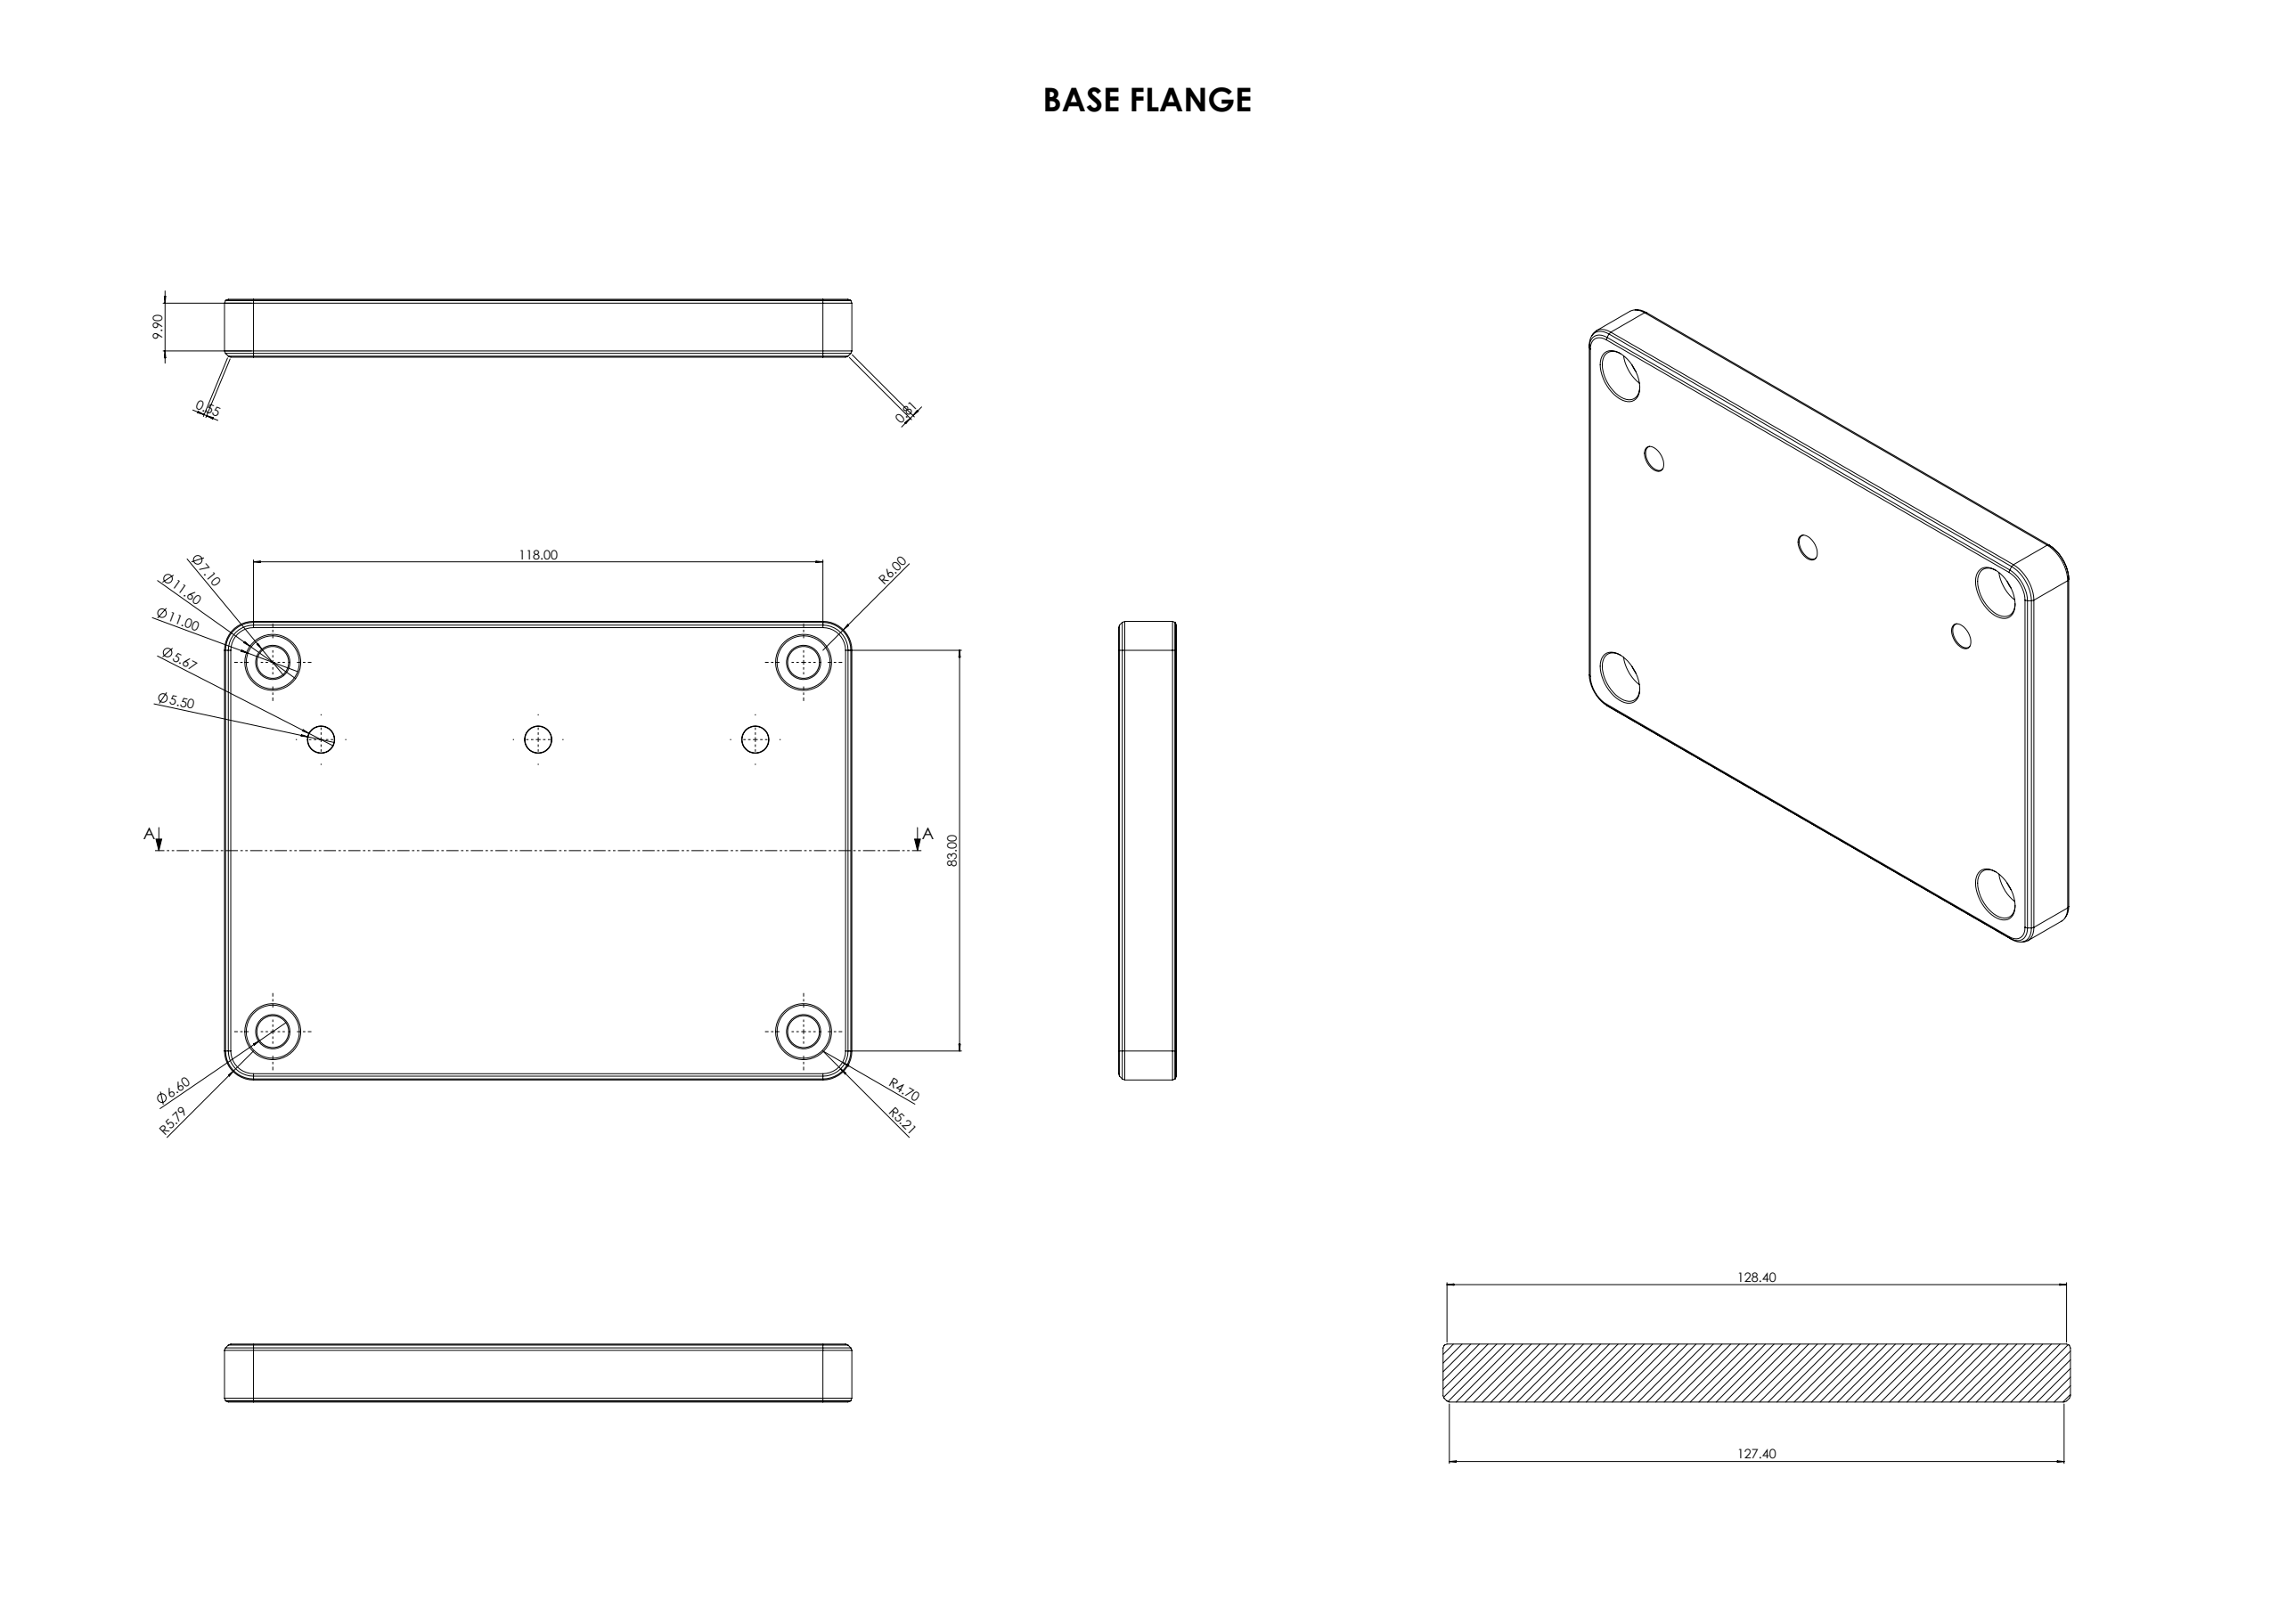
ISO-10303-21;
HEADER;
/* Generated by software containing ST-Developer
 * from STEP Tools, Inc. (www.steptools.com) 
 */

FILE_DESCRIPTION(
/* description */ (''),
/* implementation_level */ '2;1');

FILE_NAME(
/* name */ '01_Base_Flange.step',
/* time_stamp */ '2026-10-19T22:59:19-07:00',
/* author */ (''),
/* organization */ (''),
/* preprocessor_version */ 'ST-DEVELOPER v20.2',
/* originating_system */ 'Autodesk Translation Framework v15.15.0.0',
/* authorisation */ '');

FILE_SCHEMA (('AUTOMOTIVE_DESIGN { 1 0 10303 214 3 1 1 }'));
ENDSEC;

DATA;
#10=MECHANICAL_DESIGN_GEOMETRIC_PRESENTATION_REPRESENTATION('',(#911),#53650);
#879=SHAPE_REPRESENTATION_RELATIONSHIP('SRR','None',#53724,#895);
#895=ADVANCED_BREP_SHAPE_REPRESENTATION('',(#927),#53634);
#911=STYLED_ITEM('',(#53937),#927);
#927=MANIFOLD_SOLID_BREP('Base Flange',#23303);
#943=CYLINDRICAL_SURFACE('',#23543,0.6);
#944=CYLINDRICAL_SURFACE('',#23546,0.6);
#945=CYLINDRICAL_SURFACE('',#23599,0.55);
#946=CYLINDRICAL_SURFACE('',#23604,0.55);
#947=CYLINDRICAL_SURFACE('',#23609,0.55);
#948=CYLINDRICAL_SURFACE('',#23614,0.55);
#949=CYLINDRICAL_SURFACE('',#23619,0.5);
#950=CYLINDRICAL_SURFACE('',#23624,0.5);
#951=CYLINDRICAL_SURFACE('',#23629,0.5);
#952=CYLINDRICAL_SURFACE('',#23633,0.275);
#953=CYLINDRICAL_SURFACE('',#23640,0.275);
#954=CYLINDRICAL_SURFACE('',#23647,0.275);
#955=CYLINDRICAL_SURFACE('',#23654,0.33);
#956=CYLINDRICAL_SURFACE('',#23661,0.33);
#957=CYLINDRICAL_SURFACE('',#23668,0.33);
#958=CYLINDRICAL_SURFACE('',#23675,0.33);
#959=CYLINDRICAL_SURFACE('',#23683,0.6);
#960=CYLINDRICAL_SURFACE('',#23684,0.6);
#1277=FACE_BOUND('',#3577,.T.);
#1278=FACE_BOUND('',#3578,.T.);
#1279=FACE_BOUND('',#3579,.T.);
#1280=FACE_BOUND('',#3580,.T.);
#1281=FACE_BOUND('',#3581,.T.);
#1282=FACE_BOUND('',#3582,.T.);
#1283=FACE_BOUND('',#3583,.T.);
#1284=FACE_BOUND('',#3612,.T.);
#1285=FACE_BOUND('',#3613,.T.);
#1286=FACE_BOUND('',#3614,.T.);
#1287=FACE_BOUND('',#3615,.T.);
#1288=FACE_BOUND('',#3616,.T.);
#1289=FACE_BOUND('',#3617,.T.);
#1290=FACE_BOUND('',#3618,.T.);
#1291=FACE_BOUND('',#3648,.T.);
#1292=FACE_BOUND('',#3653,.T.);
#1293=FACE_BOUND('',#3658,.T.);
#1294=FACE_BOUND('',#3663,.T.);
#1295=FACE_BOUND('',#3668,.T.);
#1296=FACE_BOUND('',#3673,.T.);
#1297=FACE_BOUND('',#3678,.T.);
#1448=PLANE('',#23501);
#1449=PLANE('',#23505);
#1450=PLANE('',#23509);
#1451=PLANE('',#23513);
#1452=PLANE('',#23514);
#1453=PLANE('',#23517);
#1454=PLANE('',#23520);
#1455=PLANE('',#23530);
#1456=PLANE('',#23533);
#1457=PLANE('',#23537);
#1458=PLANE('',#23541);
#1459=PLANE('',#23542);
#1460=PLANE('',#23545);
#1461=PLANE('',#23548);
#1462=PLANE('',#23550);
#1463=PLANE('',#23551);
#1464=PLANE('',#23555);
#1465=PLANE('',#23559);
#1466=PLANE('',#23563);
#1467=PLANE('',#23569);
#1468=PLANE('',#23572);
#1469=PLANE('',#23573);
#1470=PLANE('',#23581);
#1471=PLANE('',#23583);
#1472=PLANE('',#23585);
#1473=PLANE('',#23589);
#1474=PLANE('',#23594);
#1475=PLANE('',#23637);
#1476=PLANE('',#23644);
#1477=PLANE('',#23651);
#1478=PLANE('',#23658);
#1479=PLANE('',#23665);
#1480=PLANE('',#23672);
#1481=PLANE('',#23679);
#1482=PLANE('',#23680);
#1483=PLANE('',#23682);
#1484=PLANE('',#23685);
#2236=FACE_OUTER_BOUND('',#3564,.T.);
#2237=FACE_OUTER_BOUND('',#3565,.T.);
#2238=FACE_OUTER_BOUND('',#3566,.T.);
#2239=FACE_OUTER_BOUND('',#3567,.T.);
#2240=FACE_OUTER_BOUND('',#3568,.T.);
#2241=FACE_OUTER_BOUND('',#3569,.T.);
#2242=FACE_OUTER_BOUND('',#3570,.T.);
#2243=FACE_OUTER_BOUND('',#3571,.T.);
#2244=FACE_OUTER_BOUND('',#3572,.T.);
#2245=FACE_OUTER_BOUND('',#3573,.T.);
#2246=FACE_OUTER_BOUND('',#3574,.T.);
#2247=FACE_OUTER_BOUND('',#3575,.T.);
#2248=FACE_OUTER_BOUND('',#3576,.T.);
#2249=FACE_OUTER_BOUND('',#3584,.T.);
#2250=FACE_OUTER_BOUND('',#3585,.T.);
#2251=FACE_OUTER_BOUND('',#3586,.T.);
#2252=FACE_OUTER_BOUND('',#3587,.T.);
#2253=FACE_OUTER_BOUND('',#3588,.T.);
#2254=FACE_OUTER_BOUND('',#3589,.T.);
#2255=FACE_OUTER_BOUND('',#3590,.T.);
#2256=FACE_OUTER_BOUND('',#3591,.T.);
#2257=FACE_OUTER_BOUND('',#3592,.T.);
#2258=FACE_OUTER_BOUND('',#3593,.T.);
#2259=FACE_OUTER_BOUND('',#3594,.T.);
#2260=FACE_OUTER_BOUND('',#3595,.T.);
#2261=FACE_OUTER_BOUND('',#3596,.T.);
#2262=FACE_OUTER_BOUND('',#3597,.T.);
#2263=FACE_OUTER_BOUND('',#3598,.T.);
#2264=FACE_OUTER_BOUND('',#3599,.T.);
#2265=FACE_OUTER_BOUND('',#3600,.T.);
#2266=FACE_OUTER_BOUND('',#3601,.T.);
#2267=FACE_OUTER_BOUND('',#3602,.T.);
#2268=FACE_OUTER_BOUND('',#3603,.T.);
#2269=FACE_OUTER_BOUND('',#3604,.T.);
#2270=FACE_OUTER_BOUND('',#3605,.T.);
#2271=FACE_OUTER_BOUND('',#3606,.T.);
#2272=FACE_OUTER_BOUND('',#3607,.T.);
#2273=FACE_OUTER_BOUND('',#3608,.T.);
#2274=FACE_OUTER_BOUND('',#3609,.T.);
#2275=FACE_OUTER_BOUND('',#3610,.T.);
#2276=FACE_OUTER_BOUND('',#3611,.T.);
#2277=FACE_OUTER_BOUND('',#3619,.T.);
#2278=FACE_OUTER_BOUND('',#3620,.T.);
#2279=FACE_OUTER_BOUND('',#3621,.T.);
#2280=FACE_OUTER_BOUND('',#3622,.T.);
#2281=FACE_OUTER_BOUND('',#3623,.T.);
#2282=FACE_OUTER_BOUND('',#3624,.T.);
#2283=FACE_OUTER_BOUND('',#3625,.T.);
#2284=FACE_OUTER_BOUND('',#3626,.T.);
#2285=FACE_OUTER_BOUND('',#3627,.T.);
#2286=FACE_OUTER_BOUND('',#3628,.T.);
#2287=FACE_OUTER_BOUND('',#3629,.T.);
#2288=FACE_OUTER_BOUND('',#3630,.T.);
#2289=FACE_OUTER_BOUND('',#3631,.T.);
#2290=FACE_OUTER_BOUND('',#3632,.T.);
#2291=FACE_OUTER_BOUND('',#3633,.T.);
#2292=FACE_OUTER_BOUND('',#3634,.T.);
#2293=FACE_OUTER_BOUND('',#3635,.T.);
#2294=FACE_OUTER_BOUND('',#3636,.T.);
#2295=FACE_OUTER_BOUND('',#3637,.T.);
#2296=FACE_OUTER_BOUND('',#3638,.T.);
#2297=FACE_OUTER_BOUND('',#3639,.T.);
#2298=FACE_OUTER_BOUND('',#3640,.T.);
#2299=FACE_OUTER_BOUND('',#3641,.T.);
#2300=FACE_OUTER_BOUND('',#3642,.T.);
#2301=FACE_OUTER_BOUND('',#3643,.T.);
#2302=FACE_OUTER_BOUND('',#3644,.T.);
#2303=FACE_OUTER_BOUND('',#3645,.T.);
#2304=FACE_OUTER_BOUND('',#3646,.T.);
#2305=FACE_OUTER_BOUND('',#3647,.T.);
#2306=FACE_OUTER_BOUND('',#3649,.T.);
#2307=FACE_OUTER_BOUND('',#3650,.T.);
#2308=FACE_OUTER_BOUND('',#3651,.T.);
#2309=FACE_OUTER_BOUND('',#3652,.T.);
#2310=FACE_OUTER_BOUND('',#3654,.T.);
#2311=FACE_OUTER_BOUND('',#3655,.T.);
#2312=FACE_OUTER_BOUND('',#3656,.T.);
#2313=FACE_OUTER_BOUND('',#3657,.T.);
#2314=FACE_OUTER_BOUND('',#3659,.T.);
#2315=FACE_OUTER_BOUND('',#3660,.T.);
#2316=FACE_OUTER_BOUND('',#3661,.T.);
#2317=FACE_OUTER_BOUND('',#3662,.T.);
#2318=FACE_OUTER_BOUND('',#3664,.T.);
#2319=FACE_OUTER_BOUND('',#3665,.T.);
#2320=FACE_OUTER_BOUND('',#3666,.T.);
#2321=FACE_OUTER_BOUND('',#3667,.T.);
#2322=FACE_OUTER_BOUND('',#3669,.T.);
#2323=FACE_OUTER_BOUND('',#3670,.T.);
#2324=FACE_OUTER_BOUND('',#3671,.T.);
#2325=FACE_OUTER_BOUND('',#3672,.T.);
#2326=FACE_OUTER_BOUND('',#3674,.T.);
#2327=FACE_OUTER_BOUND('',#3675,.T.);
#2328=FACE_OUTER_BOUND('',#3676,.T.);
#2329=FACE_OUTER_BOUND('',#3677,.T.);
#2330=FACE_OUTER_BOUND('',#3679,.T.);
#2331=FACE_OUTER_BOUND('',#3680,.T.);
#2332=FACE_OUTER_BOUND('',#3681,.T.);
#2333=FACE_OUTER_BOUND('',#3682,.T.);
#2334=FACE_OUTER_BOUND('',#3683,.T.);
#2335=FACE_OUTER_BOUND('',#3684,.T.);
#3564=EDGE_LOOP('',(#15067,#15068,#15069,#15070));
#3565=EDGE_LOOP('',(#15071,#15072,#15073,#15074));
#3566=EDGE_LOOP('',(#15075,#15076,#15077,#15078));
#3567=EDGE_LOOP('',(#15079,#15080,#15081,#15082));
#3568=EDGE_LOOP('',(#15083,#15084,#15085,#15086));
#3569=EDGE_LOOP('',(#15087,#15088,#15089,#15090));
#3570=EDGE_LOOP('',(#15091,#15092,#15093,#15094));
#3571=EDGE_LOOP('',(#15095,#15096,#15097,#15098));
#3572=EDGE_LOOP('',(#15099,#15100,#15101,#15102));
#3573=EDGE_LOOP('',(#15103,#15104,#15105,#15106));
#3574=EDGE_LOOP('',(#15107,#15108,#15109,#15110));
#3575=EDGE_LOOP('',(#15111,#15112,#15113,#15114));
#3576=EDGE_LOOP('',(#15115,#15116,#15117,#15118,#15119,#15120,#15121,#15122));
#3577=EDGE_LOOP('',(#15123));
#3578=EDGE_LOOP('',(#15124));
#3579=EDGE_LOOP('',(#15125));
#3580=EDGE_LOOP('',(#15126));
#3581=EDGE_LOOP('',(#15127));
#3582=EDGE_LOOP('',(#15128));
#3583=EDGE_LOOP('',(#15129));
#3584=EDGE_LOOP('',(#15130,#15131,#15132,#15133));
#3585=EDGE_LOOP('',(#15134,#15135,#15136,#15137));
#3586=EDGE_LOOP('',(#15138,#15139,#15140,#15141));
#3587=EDGE_LOOP('',(#15142,#15143,#15144,#15145));
#3588=EDGE_LOOP('',(#15146,#15147,#15148,#15149));
#3589=EDGE_LOOP('',(#15150,#15151,#15152,#15153));
#3590=EDGE_LOOP('',(#15154,#15155,#15156,#15157));
#3591=EDGE_LOOP('',(#15158,#15159,#15160,#15161));
#3592=EDGE_LOOP('',(#15162,#15163,#15164,#15165));
#3593=EDGE_LOOP('',(#15166,#15167,#15168,#15169));
#3594=EDGE_LOOP('',(#15170,#15171,#15172,#15173));
#3595=EDGE_LOOP('',(#15174,#15175,#15176,#15177));
#3596=EDGE_LOOP('',(#15178,#15179,#15180,#15181));
#3597=EDGE_LOOP('',(#15182,#15183,#15184,#15185));
#3598=EDGE_LOOP('',(#15186,#15187,#15188,#15189));
#3599=EDGE_LOOP('',(#15190,#15191,#15192,#15193));
#3600=EDGE_LOOP('',(#15194,#15195,#15196,#15197));
#3601=EDGE_LOOP('',(#15198,#15199,#15200,#15201));
#3602=EDGE_LOOP('',(#15202,#15203,#15204,#15205));
#3603=EDGE_LOOP('',(#15206,#15207,#15208,#15209));
#3604=EDGE_LOOP('',(#15210,#15211,#15212,#15213));
#3605=EDGE_LOOP('',(#15214,#15215,#15216,#15217));
#3606=EDGE_LOOP('',(#15218,#15219,#15220,#15221));
#3607=EDGE_LOOP('',(#15222,#15223,#15224,#15225));
#3608=EDGE_LOOP('',(#15226,#15227,#15228,#15229));
#3609=EDGE_LOOP('',(#15230,#15231,#15232,#15233));
#3610=EDGE_LOOP('',(#15234,#15235,#15236,#15237));
#3611=EDGE_LOOP('',(#15238,#15239,#15240,#15241,#15242,#15243,#15244,#15245));
#3612=EDGE_LOOP('',(#15246));
#3613=EDGE_LOOP('',(#15247));
#3614=EDGE_LOOP('',(#15248));
#3615=EDGE_LOOP('',(#15249));
#3616=EDGE_LOOP('',(#15250));
#3617=EDGE_LOOP('',(#15251));
#3618=EDGE_LOOP('',(#15252));
#3619=EDGE_LOOP('',(#15253,#15254,#15255,#15256));
#3620=EDGE_LOOP('',(#15257,#15258,#15259,#15260));
#3621=EDGE_LOOP('',(#15261,#15262,#15263,#15264));
#3622=EDGE_LOOP('',(#15265,#15266,#15267,#15268));
#3623=EDGE_LOOP('',(#15269,#15270,#15271,#15272));
#3624=EDGE_LOOP('',(#15273,#15274,#15275,#15276));
#3625=EDGE_LOOP('',(#15277,#15278,#15279,#15280));
#3626=EDGE_LOOP('',(#15281,#15282,#15283,#15284));
#3627=EDGE_LOOP('',(#15285,#15286,#15287,#15288));
#3628=EDGE_LOOP('',(#15289,#15290,#15291,#15292));
#3629=EDGE_LOOP('',(#15293,#15294,#15295,#15296));
#3630=EDGE_LOOP('',(#15297,#15298,#15299,#15300,#15301));
#3631=EDGE_LOOP('',(#15302,#15303,#15304,#15305,#15306));
#3632=EDGE_LOOP('',(#15307,#15308,#15309,#15310,#15311));
#3633=EDGE_LOOP('',(#15312,#15313,#15314,#15315,#15316));
#3634=EDGE_LOOP('',(#15317,#15318,#15319,#15320,#15321));
#3635=EDGE_LOOP('',(#15322,#15323,#15324,#15325,#15326));
#3636=EDGE_LOOP('',(#15327,#15328,#15329,#15330,#15331));
#3637=EDGE_LOOP('',(#15332,#15333,#15334,#15335,#15336));
#3638=EDGE_LOOP('',(#15337,#15338,#15339,#15340,#15341));
#3639=EDGE_LOOP('',(#15342,#15343,#15344,#15345,#15346));
#3640=EDGE_LOOP('',(#15347,#15348,#15349,#15350,#15351));
#3641=EDGE_LOOP('',(#15352,#15353,#15354,#15355,#15356));
#3642=EDGE_LOOP('',(#15357,#15358,#15359,#15360,#15361));
#3643=EDGE_LOOP('',(#15362,#15363,#15364,#15365,#15366));
#3644=EDGE_LOOP('',(#15367,#15368,#15369,#15370));
#3645=EDGE_LOOP('',(#15371,#15372,#15373,#15374));
#3646=EDGE_LOOP('',(#15375,#15376,#15377,#15378));
#3647=EDGE_LOOP('',(#15379));
#3648=EDGE_LOOP('',(#15380));
#3649=EDGE_LOOP('',(#15381,#15382,#15383,#15384));
#3650=EDGE_LOOP('',(#15385,#15386,#15387,#15388));
#3651=EDGE_LOOP('',(#15389,#15390,#15391,#15392));
#3652=EDGE_LOOP('',(#15393));
#3653=EDGE_LOOP('',(#15394));
#3654=EDGE_LOOP('',(#15395,#15396,#15397,#15398));
#3655=EDGE_LOOP('',(#15399,#15400,#15401,#15402));
#3656=EDGE_LOOP('',(#15403,#15404,#15405,#15406));
#3657=EDGE_LOOP('',(#15407));
#3658=EDGE_LOOP('',(#15408));
#3659=EDGE_LOOP('',(#15409,#15410,#15411,#15412));
#3660=EDGE_LOOP('',(#15413,#15414,#15415,#15416));
#3661=EDGE_LOOP('',(#15417,#15418,#15419,#15420));
#3662=EDGE_LOOP('',(#15421));
#3663=EDGE_LOOP('',(#15422));
#3664=EDGE_LOOP('',(#15423,#15424,#15425,#15426));
#3665=EDGE_LOOP('',(#15427,#15428,#15429,#15430));
#3666=EDGE_LOOP('',(#15431,#15432,#15433,#15434));
#3667=EDGE_LOOP('',(#15435));
#3668=EDGE_LOOP('',(#15436));
#3669=EDGE_LOOP('',(#15437,#15438,#15439,#15440));
#3670=EDGE_LOOP('',(#15441,#15442,#15443,#15444));
#3671=EDGE_LOOP('',(#15445,#15446,#15447,#15448));
#3672=EDGE_LOOP('',(#15449));
#3673=EDGE_LOOP('',(#15450));
#3674=EDGE_LOOP('',(#15451,#15452,#15453,#15454));
#3675=EDGE_LOOP('',(#15455,#15456,#15457,#15458));
#3676=EDGE_LOOP('',(#15459,#15460,#15461,#15462));
#3677=EDGE_LOOP('',(#15463));
#3678=EDGE_LOOP('',(#15464));
#3679=EDGE_LOOP('',(#15465,#15466,#15467,#15468));
#3680=EDGE_LOOP('',(#15469,#15470,#15471,#15472));
#3681=EDGE_LOOP('',(#15473,#15474,#15475,#15476));
#3682=EDGE_LOOP('',(#15477,#15478,#15479,#15480));
#3683=EDGE_LOOP('',(#15481,#15482,#15483,#15484));
#3684=EDGE_LOOP('',(#15485,#15486,#15487,#15488));
#5063=CIRCLE('',#23499,0.521213203435596);
#5064=CIRCLE('',#23500,0.47);
#5065=CIRCLE('',#23503,0.521213203435596);
#5066=CIRCLE('',#23504,0.47);
#5067=CIRCLE('',#23507,0.521213203435596);
#5068=CIRCLE('',#23508,0.47);
#5069=CIRCLE('',#23511,0.521213203435596);
#5070=CIRCLE('',#23512,0.47);
#5071=CIRCLE('',#23516,0.578786796564404);
#5072=CIRCLE('',#23519,0.578786796564404);
#5073=CIRCLE('',#23521,0.58);
#5074=CIRCLE('',#23522,0.58);
#5075=CIRCLE('',#23523,0.283333333333333);
#5076=CIRCLE('',#23524,0.283333333333333);
#5077=CIRCLE('',#23525,0.283333333333333);
#5078=CIRCLE('',#23526,0.58);
#5079=CIRCLE('',#23527,0.58);
#5080=CIRCLE('',#23529,0.6);
#5081=CIRCLE('',#23532,0.6);
#5082=CIRCLE('',#23535,0.578786796564404);
#5083=CIRCLE('',#23536,0.6);
#5084=CIRCLE('',#23539,0.578786796564404);
#5085=CIRCLE('',#23540,0.6);
#5086=CIRCLE('',#23544,0.6);
#5087=CIRCLE('',#23547,0.6);
#5088=CIRCLE('',#23553,0.571213203435596);
#5089=CIRCLE('',#23554,0.52);
#5090=CIRCLE('',#23557,0.571213203435596);
#5091=CIRCLE('',#23558,0.52);
#5092=CIRCLE('',#23561,0.571213203435596);
#5093=CIRCLE('',#23562,0.52);
#5094=CIRCLE('',#23565,0.571213203435596);
#5095=CIRCLE('',#23566,0.52);
#5096=CIRCLE('',#23568,0.578786796564404);
#5097=CIRCLE('',#23571,0.578786796564404);
#5098=CIRCLE('',#23574,0.53);
#5099=CIRCLE('',#23575,0.53);
#5100=CIRCLE('',#23576,0.338333333333333);
#5101=CIRCLE('',#23577,0.338333333333333);
#5102=CIRCLE('',#23578,0.338333333333333);
#5103=CIRCLE('',#23579,0.338333333333333);
#5104=CIRCLE('',#23580,0.53);
#5105=CIRCLE('',#23587,0.578786796564404);
#5106=CIRCLE('',#23588,0.6);
#5107=CIRCLE('',#23591,0.578786796564404);
#5108=CIRCLE('',#23592,0.6);
#5109=CIRCLE('',#23597,0.55);
#5110=CIRCLE('',#23598,0.55);
#5111=CIRCLE('',#23600,0.55);
#5112=CIRCLE('',#23602,0.55);
#5113=CIRCLE('',#23603,0.55);
#5114=CIRCLE('',#23605,0.55);
#5115=CIRCLE('',#23607,0.55);
#5116=CIRCLE('',#23608,0.55);
#5117=CIRCLE('',#23610,0.55);
#5118=CIRCLE('',#23612,0.55);
#5119=CIRCLE('',#23613,0.55);
#5120=CIRCLE('',#23615,0.55);
#5121=CIRCLE('',#23617,0.5);
#5122=CIRCLE('',#23618,0.5);
#5123=CIRCLE('',#23620,0.5);
#5124=CIRCLE('',#23622,0.5);
#5125=CIRCLE('',#23623,0.5);
#5126=CIRCLE('',#23625,0.5);
#5127=CIRCLE('',#23627,0.5);
#5128=CIRCLE('',#23628,0.5);
#5129=CIRCLE('',#23630,0.5);
#5130=CIRCLE('',#23632,0.275);
#5131=CIRCLE('',#23634,0.275);
#5132=CIRCLE('',#23636,0.3);
#5133=CIRCLE('',#23639,0.275);
#5134=CIRCLE('',#23641,0.275);
#5135=CIRCLE('',#23643,0.3);
#5136=CIRCLE('',#23646,0.275);
#5137=CIRCLE('',#23648,0.275);
#5138=CIRCLE('',#23650,0.3);
#5139=CIRCLE('',#23653,0.33);
#5140=CIRCLE('',#23655,0.33);
#5141=CIRCLE('',#23657,0.355);
#5142=CIRCLE('',#23660,0.33);
#5143=CIRCLE('',#23662,0.33);
#5144=CIRCLE('',#23664,0.355);
#5145=CIRCLE('',#23667,0.33);
#5146=CIRCLE('',#23669,0.33);
#5147=CIRCLE('',#23671,0.355);
#5148=CIRCLE('',#23674,0.33);
#5149=CIRCLE('',#23676,0.33);
#5150=CIRCLE('',#23678,0.355);
#5852=LINE('',#31820,#7697);
#5853=LINE('',#31824,#7698);
#5854=LINE('',#31829,#7699);
#5855=LINE('',#31830,#7700);
#5856=LINE('',#31831,#7701);
#5857=LINE('',#31835,#7702);
#5858=LINE('',#31841,#7703);
#5859=LINE('',#31842,#7704);
#5860=LINE('',#31843,#7705);
#5861=LINE('',#31847,#7706);
#5862=LINE('',#31853,#7707);
#5863=LINE('',#31854,#7708);
#5864=LINE('',#31855,#7709);
#5865=LINE('',#31859,#7710);
#5866=LINE('',#31863,#7711);
#5867=LINE('',#31864,#7712);
#5868=LINE('',#31867,#7713);
#5869=LINE('',#31869,#7714);
#5870=LINE('',#31870,#7715);
#5871=LINE('',#31873,#7716);
#5872=LINE('',#31877,#7717);
#5873=LINE('',#31878,#7718);
#5874=LINE('',#31881,#7719);
#5875=LINE('',#31900,#7720);
#5876=LINE('',#31902,#7721);
#5877=LINE('',#31906,#7722);
#5878=LINE('',#31907,#7723);
#5879=LINE('',#31910,#7724);
#5880=LINE('',#31914,#7725);
#5881=LINE('',#31915,#7726);
#5882=LINE('',#31919,#7727);
#5883=LINE('',#31925,#7728);
#5884=LINE('',#31926,#7729);
#5885=LINE('',#31927,#7730);
#5886=LINE('',#31931,#7731);
#5887=LINE('',#31935,#7732);
#5888=LINE('',#31936,#7733);
#5889=LINE('',#31939,#7734);
#5890=LINE('',#31941,#7735);
#5891=LINE('',#31942,#7736);
#5892=LINE('',#31945,#7737);
#5893=LINE('',#31949,#7738);
#5894=LINE('',#31950,#7739);
#5895=LINE('',#31953,#7740);
#5896=LINE('',#31956,#7741);
#5897=LINE('',#31957,#7742);
#5898=LINE('',#31959,#7743);
#5899=LINE('',#31964,#7744);
#5900=LINE('',#31966,#7745);
#5901=LINE('',#31968,#7746);
#5902=LINE('',#31969,#7747);
#5903=LINE('',#31973,#7748);
#5904=LINE('',#31979,#7749);
#5905=LINE('',#31980,#7750);
#5906=LINE('',#31981,#7751);
#5907=LINE('',#31985,#7752);
#5908=LINE('',#31991,#7753);
#5909=LINE('',#31992,#7754);
#5910=LINE('',#31993,#7755);
#5911=LINE('',#31997,#7756);
#5912=LINE('',#32003,#7757);
#5913=LINE('',#32004,#7758);
#5914=LINE('',#32005,#7759);
#5915=LINE('',#32011,#7760);
#5916=LINE('',#32014,#7761);
#5917=LINE('',#32017,#7762);
#5918=LINE('',#32018,#7763);
#5919=LINE('',#32021,#7764);
#5920=LINE('',#32025,#7765);
#5921=LINE('',#32026,#7766);
#5922=LINE('',#32043,#7767);
#5923=LINE('',#32044,#7768);
#5924=LINE('',#32046,#7769);
#5925=LINE('',#32048,#7770);
#5926=LINE('',#32050,#7771);
#5927=LINE('',#32054,#7772);
#5928=LINE('',#32055,#7773);
#5929=LINE('',#32056,#7774);
#5930=LINE('',#32060,#7775);
#5931=LINE('',#32066,#7776);
#5932=LINE('',#32067,#7777);
#5933=LINE('',#32068,#7778);
#5934=LINE('',#32073,#7779);
#5935=LINE('',#32074,#7780);
#5936=LINE('',#32076,#7781);
#5937=LINE('',#32080,#7782);
#5938=LINE('',#32087,#7783);
#5939=LINE('',#32090,#7784);
#5940=LINE('',#32097,#7785);
#5941=LINE('',#32100,#7786);
#5942=LINE('',#32107,#7787);
#5943=LINE('',#32110,#7788);
#5944=LINE('',#32117,#7789);
#5945=LINE('',#32120,#7790);
#5946=LINE('',#32127,#7791);
#5947=LINE('',#32130,#7792);
#5948=LINE('',#32137,#7793);
#5949=LINE('',#32140,#7794);
#5950=LINE('',#32147,#7795);
#5951=LINE('',#32150,#7796);
#5952=LINE('',#32154,#7797);
#5953=LINE('',#32158,#7798);
#5954=LINE('',#32163,#7799);
#5955=LINE('',#32167,#7800);
#5956=LINE('',#32171,#7801);
#5957=LINE('',#32176,#7802);
#5958=LINE('',#32180,#7803);
#5959=LINE('',#32184,#7804);
#5960=LINE('',#32189,#7805);
#5961=LINE('',#32193,#7806);
#5962=LINE('',#32197,#7807);
#5963=LINE('',#32202,#7808);
#5964=LINE('',#32206,#7809);
#5965=LINE('',#32210,#7810);
#5966=LINE('',#32215,#7811);
#5967=LINE('',#32219,#7812);
#5968=LINE('',#32223,#7813);
#5969=LINE('',#32228,#7814);
#5970=LINE('',#32232,#7815);
#5971=LINE('',#32236,#7816);
#5972=LINE('',#32242,#7817);
#5973=LINE('',#32244,#7818);
#5974=LINE('',#32246,#7819);
#7697=VECTOR('',#25660,1.);
#7698=VECTOR('',#25663,1.);
#7699=VECTOR('',#25668,1.);
#7700=VECTOR('',#25669,1.);
#7701=VECTOR('',#25670,1.);
#7702=VECTOR('',#25673,1.);
#7703=VECTOR('',#25680,1.);
#7704=VECTOR('',#25681,1.);
#7705=VECTOR('',#25682,1.);
#7706=VECTOR('',#25685,1.);
#7707=VECTOR('',#25692,1.);
#7708=VECTOR('',#25693,1.);
#7709=VECTOR('',#25694,1.);
#7710=VECTOR('',#25697,1.);
#7711=VECTOR('',#25704,1.);
#7712=VECTOR('',#25705,1.);
#7713=VECTOR('',#25708,1.);
#7714=VECTOR('',#25709,1.);
#7715=VECTOR('',#25710,1.);
#7716=VECTOR('',#25713,1.);
#7717=VECTOR('',#25718,1.);
#7718=VECTOR('',#25719,1.);
#7719=VECTOR('',#25722,1.);
#7720=VECTOR('',#25743,1.);
#7721=VECTOR('',#25744,1.);
#7722=VECTOR('',#25749,1.);
#7723=VECTOR('',#25750,1.);
#7724=VECTOR('',#25753,1.);
#7725=VECTOR('',#25758,1.);
#7726=VECTOR('',#25759,1.);
#7727=VECTOR('',#25762,1.);
#7728=VECTOR('',#25769,1.);
#7729=VECTOR('',#25770,1.);
#7730=VECTOR('',#25771,1.);
#7731=VECTOR('',#25774,1.);
#7732=VECTOR('',#25781,1.);
#7733=VECTOR('',#25782,1.);
#7734=VECTOR('',#25785,1.);
#7735=VECTOR('',#25786,1.);
#7736=VECTOR('',#25787,1.);
#7737=VECTOR('',#25790,1.);
#7738=VECTOR('',#25795,1.);
#7739=VECTOR('',#25796,1.);
#7740=VECTOR('',#25799,1.);
#7741=VECTOR('',#25804,1.);
#7742=VECTOR('',#25805,1.);
#7743=VECTOR('',#25808,1.);
#7744=VECTOR('',#25813,1.);
#7745=VECTOR('',#25814,1.);
#7746=VECTOR('',#25815,1.);
#7747=VECTOR('',#25816,1.);
#7748=VECTOR('',#25819,1.);
#7749=VECTOR('',#25826,1.);
#7750=VECTOR('',#25827,1.);
#7751=VECTOR('',#25828,1.);
#7752=VECTOR('',#25831,1.);
#7753=VECTOR('',#25838,1.);
#7754=VECTOR('',#25839,1.);
#7755=VECTOR('',#25840,1.);
#7756=VECTOR('',#25843,1.);
#7757=VECTOR('',#25850,1.);
#7758=VECTOR('',#25851,1.);
#7759=VECTOR('',#25852,1.);
#7760=VECTOR('',#25861,1.);
#7761=VECTOR('',#25864,1.);
#7762=VECTOR('',#25867,1.);
#7763=VECTOR('',#25868,1.);
#7764=VECTOR('',#25871,1.);
#7765=VECTOR('',#25876,1.);
#7766=VECTOR('',#25877,1.);
#7767=VECTOR('',#25896,1.);
#7768=VECTOR('',#25897,1.);
#7769=VECTOR('',#25900,1.);
#7770=VECTOR('',#25903,1.);
#7771=VECTOR('',#25906,1.);
#7772=VECTOR('',#25909,1.);
#7773=VECTOR('',#25910,1.);
#7774=VECTOR('',#25911,1.);
#7775=VECTOR('',#25914,1.);
#7776=VECTOR('',#25921,1.);
#7777=VECTOR('',#25922,1.);
#7778=VECTOR('',#25923,1.);
#7779=VECTOR('',#25932,1.);
#7780=VECTOR('',#25933,1.);
#7781=VECTOR('',#25936,1.);
#7782=VECTOR('',#25941,0.565);
#7783=VECTOR('',#25950,0.55);
#7784=VECTOR('',#25953,0.565);
#7785=VECTOR('',#25962,0.55);
#7786=VECTOR('',#25965,0.565);
#7787=VECTOR('',#25974,0.55);
#7788=VECTOR('',#25977,0.565);
#7789=VECTOR('',#25986,0.55);
#7790=VECTOR('',#25989,0.515);
#7791=VECTOR('',#25998,0.5);
#7792=VECTOR('',#26001,0.515);
#7793=VECTOR('',#26010,0.5);
#7794=VECTOR('',#26013,0.515);
#7795=VECTOR('',#26022,0.5);
#7796=VECTOR('',#26025,0.2875);
#7797=VECTOR('',#26030,0.275);
#7798=VECTOR('',#26035,0.2875);
#7799=VECTOR('',#26042,0.2875);
#7800=VECTOR('',#26047,0.275);
#7801=VECTOR('',#26052,0.2875);
#7802=VECTOR('',#26059,0.2875);
#7803=VECTOR('',#26064,0.275);
#7804=VECTOR('',#26069,0.2875);
#7805=VECTOR('',#26076,0.342499999999999);
#7806=VECTOR('',#26081,0.33);
#7807=VECTOR('',#26086,0.342499999999999);
#7808=VECTOR('',#26093,0.342499999999999);
#7809=VECTOR('',#26098,0.33);
#7810=VECTOR('',#26103,0.342499999999999);
#7811=VECTOR('',#26110,0.342499999999999);
#7812=VECTOR('',#26115,0.33);
#7813=VECTOR('',#26120,0.342499999999999);
#7814=VECTOR('',#26127,0.342499999999999);
#7815=VECTOR('',#26132,0.33);
#7816=VECTOR('',#26137,0.342499999999999);
#7817=VECTOR('',#26148,1.);
#7818=VECTOR('',#26151,1.);
#7819=VECTOR('',#26154,1.);
#9542=VERTEX_POINT('',#31818);
#9543=VERTEX_POINT('',#31819);
#9544=VERTEX_POINT('',#31821);
#9545=VERTEX_POINT('',#31823);
#9546=VERTEX_POINT('',#31827);
#9547=VERTEX_POINT('',#31828);
#9548=VERTEX_POINT('',#31833);
#9549=VERTEX_POINT('',#31834);
#9550=VERTEX_POINT('',#31839);
#9551=VERTEX_POINT('',#31840);
#9552=VERTEX_POINT('',#31845);
#9553=VERTEX_POINT('',#31846);
#9554=VERTEX_POINT('',#31851);
#9555=VERTEX_POINT('',#31852);
#9556=VERTEX_POINT('',#31857);
#9557=VERTEX_POINT('',#31858);
#9558=VERTEX_POINT('',#31866);
#9559=VERTEX_POINT('',#31868);
#9560=VERTEX_POINT('',#31872);
#9561=VERTEX_POINT('',#31876);
#9562=VERTEX_POINT('',#31880);
#9563=VERTEX_POINT('',#31884);
#9564=VERTEX_POINT('',#31886);
#9565=VERTEX_POINT('',#31888);
#9566=VERTEX_POINT('',#31890);
#9567=VERTEX_POINT('',#31892);
#9568=VERTEX_POINT('',#31894);
#9569=VERTEX_POINT('',#31896);
#9570=VERTEX_POINT('',#31899);
#9571=VERTEX_POINT('',#31901);
#9572=VERTEX_POINT('',#31905);
#9573=VERTEX_POINT('',#31909);
#9574=VERTEX_POINT('',#31913);
#9575=VERTEX_POINT('',#31917);
#9576=VERTEX_POINT('',#31918);
#9577=VERTEX_POINT('',#31923);
#9578=VERTEX_POINT('',#31924);
#9579=VERTEX_POINT('',#31929);
#9580=VERTEX_POINT('',#31930);
#9581=VERTEX_POINT('',#31938);
#9582=VERTEX_POINT('',#31940);
#9583=VERTEX_POINT('',#31944);
#9584=VERTEX_POINT('',#31948);
#9585=VERTEX_POINT('',#31952);
#9586=VERTEX_POINT('',#31962);
#9587=VERTEX_POINT('',#31963);
#9588=VERTEX_POINT('',#31965);
#9589=VERTEX_POINT('',#31967);
#9590=VERTEX_POINT('',#31971);
#9591=VERTEX_POINT('',#31972);
#9592=VERTEX_POINT('',#31977);
#9593=VERTEX_POINT('',#31978);
#9594=VERTEX_POINT('',#31983);
#9595=VERTEX_POINT('',#31984);
#9596=VERTEX_POINT('',#31989);
#9597=VERTEX_POINT('',#31990);
#9598=VERTEX_POINT('',#31995);
#9599=VERTEX_POINT('',#31996);
#9600=VERTEX_POINT('',#32001);
#9601=VERTEX_POINT('',#32002);
#9602=VERTEX_POINT('',#32010);
#9603=VERTEX_POINT('',#32012);
#9604=VERTEX_POINT('',#32016);
#9605=VERTEX_POINT('',#32020);
#9606=VERTEX_POINT('',#32024);
#9607=VERTEX_POINT('',#32028);
#9608=VERTEX_POINT('',#32030);
#9609=VERTEX_POINT('',#32032);
#9610=VERTEX_POINT('',#32034);
#9611=VERTEX_POINT('',#32036);
#9612=VERTEX_POINT('',#32038);
#9613=VERTEX_POINT('',#32040);
#9614=VERTEX_POINT('',#32052);
#9615=VERTEX_POINT('',#32053);
#9616=VERTEX_POINT('',#32058);
#9617=VERTEX_POINT('',#32059);
#9618=VERTEX_POINT('',#32064);
#9619=VERTEX_POINT('',#32065);
#9620=VERTEX_POINT('',#32079);
#9621=VERTEX_POINT('',#32081);
#9622=VERTEX_POINT('',#32085);
#9623=VERTEX_POINT('',#32089);
#9624=VERTEX_POINT('',#32091);
#9625=VERTEX_POINT('',#32095);
#9626=VERTEX_POINT('',#32099);
#9627=VERTEX_POINT('',#32101);
#9628=VERTEX_POINT('',#32105);
#9629=VERTEX_POINT('',#32109);
#9630=VERTEX_POINT('',#32111);
#9631=VERTEX_POINT('',#32115);
#9632=VERTEX_POINT('',#32119);
#9633=VERTEX_POINT('',#32121);
#9634=VERTEX_POINT('',#32125);
#9635=VERTEX_POINT('',#32129);
#9636=VERTEX_POINT('',#32131);
#9637=VERTEX_POINT('',#32135);
#9638=VERTEX_POINT('',#32139);
#9639=VERTEX_POINT('',#32141);
#9640=VERTEX_POINT('',#32145);
#9641=VERTEX_POINT('',#32149);
#9642=VERTEX_POINT('',#32153);
#9643=VERTEX_POINT('',#32157);
#9644=VERTEX_POINT('',#32162);
#9645=VERTEX_POINT('',#32166);
#9646=VERTEX_POINT('',#32170);
#9647=VERTEX_POINT('',#32175);
#9648=VERTEX_POINT('',#32179);
#9649=VERTEX_POINT('',#32183);
#9650=VERTEX_POINT('',#32188);
#9651=VERTEX_POINT('',#32192);
#9652=VERTEX_POINT('',#32196);
#9653=VERTEX_POINT('',#32201);
#9654=VERTEX_POINT('',#32205);
#9655=VERTEX_POINT('',#32209);
#9656=VERTEX_POINT('',#32214);
#9657=VERTEX_POINT('',#32218);
#9658=VERTEX_POINT('',#32222);
#9659=VERTEX_POINT('',#32227);
#9660=VERTEX_POINT('',#32231);
#9661=VERTEX_POINT('',#32235);
#11711=EDGE_CURVE('',#9542,#9543,#5852,.T.);
#11712=EDGE_CURVE('',#9543,#9544,#5063,.T.);
#11713=EDGE_CURVE('',#9544,#9545,#5853,.T.);
#11714=EDGE_CURVE('',#9545,#9542,#5064,.T.);
#11715=EDGE_CURVE('',#9546,#9547,#5854,.T.);
#11716=EDGE_CURVE('',#9547,#9543,#5855,.T.);
#11717=EDGE_CURVE('',#9542,#9546,#5856,.T.);
#11718=EDGE_CURVE('',#9548,#9549,#5857,.T.);
#11719=EDGE_CURVE('',#9549,#9547,#5065,.T.);
#11720=EDGE_CURVE('',#9546,#9548,#5066,.T.);
#11721=EDGE_CURVE('',#9550,#9551,#5858,.T.);
#11722=EDGE_CURVE('',#9551,#9549,#5859,.T.);
#11723=EDGE_CURVE('',#9548,#9550,#5860,.T.);
#11724=EDGE_CURVE('',#9552,#9553,#5861,.T.);
#11725=EDGE_CURVE('',#9553,#9551,#5067,.T.);
#11726=EDGE_CURVE('',#9550,#9552,#5068,.T.);
#11727=EDGE_CURVE('',#9554,#9555,#5862,.T.);
#11728=EDGE_CURVE('',#9555,#9553,#5863,.T.);
#11729=EDGE_CURVE('',#9552,#9554,#5864,.T.);
#11730=EDGE_CURVE('',#9556,#9557,#5865,.T.);
#11731=EDGE_CURVE('',#9557,#9555,#5069,.T.);
#11732=EDGE_CURVE('',#9554,#9556,#5070,.T.);
#11733=EDGE_CURVE('',#9544,#9557,#5866,.T.);
#11734=EDGE_CURVE('',#9556,#9545,#5867,.T.);
#11735=EDGE_CURVE('',#9555,#9558,#5868,.T.);
#11736=EDGE_CURVE('',#9559,#9558,#5869,.T.);
#11737=EDGE_CURVE('',#9553,#9559,#5870,.T.);
#11738=EDGE_CURVE('',#9557,#9560,#5871,.T.);
#11739=EDGE_CURVE('',#9558,#9560,#5071,.T.);
#11740=EDGE_CURVE('',#9561,#9544,#5872,.T.);
#11741=EDGE_CURVE('',#9560,#9561,#5873,.T.);
#11742=EDGE_CURVE('',#9543,#9562,#5874,.T.);
#11743=EDGE_CURVE('',#9561,#9562,#5072,.T.);
#11744=EDGE_CURVE('',#9563,#9563,#5073,.T.);
#11745=EDGE_CURVE('',#9564,#9564,#5074,.T.);
#11746=EDGE_CURVE('',#9565,#9565,#5075,.T.);
#11747=EDGE_CURVE('',#9566,#9566,#5076,.T.);
#11748=EDGE_CURVE('',#9567,#9567,#5077,.T.);
#11749=EDGE_CURVE('',#9568,#9568,#5078,.T.);
#11750=EDGE_CURVE('',#9569,#9569,#5079,.T.);
#11751=EDGE_CURVE('',#9570,#9561,#5875,.T.);
#11752=EDGE_CURVE('',#9562,#9571,#5876,.T.);
#11753=EDGE_CURVE('',#9571,#9570,#5080,.T.);
#11754=EDGE_CURVE('',#9572,#9560,#5877,.T.);
#11755=EDGE_CURVE('',#9570,#9572,#5878,.T.);
#11756=EDGE_CURVE('',#9573,#9558,#5879,.T.);
#11757=EDGE_CURVE('',#9572,#9573,#5081,.T.);
#11758=EDGE_CURVE('',#9574,#9559,#5880,.T.);
#11759=EDGE_CURVE('',#9573,#9574,#5881,.T.);
#11760=EDGE_CURVE('',#9575,#9576,#5882,.T.);
#11761=EDGE_CURVE('',#9576,#9559,#5082,.T.);
#11762=EDGE_CURVE('',#9574,#9575,#5083,.T.);
#11763=EDGE_CURVE('',#9577,#9578,#5883,.T.);
#11764=EDGE_CURVE('',#9578,#9576,#5884,.T.);
#11765=EDGE_CURVE('',#9575,#9577,#5885,.T.);
#11766=EDGE_CURVE('',#9579,#9580,#5886,.T.);
#11767=EDGE_CURVE('',#9580,#9578,#5084,.T.);
#11768=EDGE_CURVE('',#9577,#9579,#5085,.T.);
#11769=EDGE_CURVE('',#9562,#9580,#5887,.T.);
#11770=EDGE_CURVE('',#9579,#9571,#5888,.T.);
#11771=EDGE_CURVE('',#9581,#9573,#5889,.T.);
#11772=EDGE_CURVE('',#9582,#9581,#5890,.T.);
#11773=EDGE_CURVE('',#9574,#9582,#5891,.T.);
#11774=EDGE_CURVE('',#9572,#9583,#5892,.T.);
#11775=EDGE_CURVE('',#9581,#9583,#5086,.T.);
#11776=EDGE_CURVE('',#9584,#9570,#5893,.T.);
#11777=EDGE_CURVE('',#9583,#9584,#5894,.T.);
#11778=EDGE_CURVE('',#9571,#9585,#5895,.T.);
#11779=EDGE_CURVE('',#9584,#9585,#5087,.T.);
#11780=EDGE_CURVE('',#9551,#9576,#5896,.T.);
#11781=EDGE_CURVE('',#9549,#9578,#5897,.T.);
#11782=EDGE_CURVE('',#9547,#9580,#5898,.T.);
#11783=EDGE_CURVE('',#9586,#9587,#5899,.T.);
#11784=EDGE_CURVE('',#9587,#9588,#5900,.T.);
#11785=EDGE_CURVE('',#9588,#9589,#5901,.T.);
#11786=EDGE_CURVE('',#9589,#9586,#5902,.T.);
#11787=EDGE_CURVE('',#9590,#9591,#5903,.T.);
#11788=EDGE_CURVE('',#9591,#9587,#5088,.T.);
#11789=EDGE_CURVE('',#9586,#9590,#5089,.T.);
#11790=EDGE_CURVE('',#9592,#9593,#5904,.T.);
#11791=EDGE_CURVE('',#9593,#9591,#5905,.T.);
#11792=EDGE_CURVE('',#9590,#9592,#5906,.T.);
#11793=EDGE_CURVE('',#9594,#9595,#5907,.T.);
#11794=EDGE_CURVE('',#9595,#9593,#5090,.T.);
#11795=EDGE_CURVE('',#9592,#9594,#5091,.T.);
#11796=EDGE_CURVE('',#9596,#9597,#5908,.T.);
#11797=EDGE_CURVE('',#9597,#9595,#5909,.T.);
#11798=EDGE_CURVE('',#9594,#9596,#5910,.T.);
#11799=EDGE_CURVE('',#9598,#9599,#5911,.T.);
#11800=EDGE_CURVE('',#9599,#9597,#5092,.T.);
#11801=EDGE_CURVE('',#9596,#9598,#5093,.T.);
#11802=EDGE_CURVE('',#9600,#9601,#5912,.T.);
#11803=EDGE_CURVE('',#9601,#9599,#5913,.T.);
#11804=EDGE_CURVE('',#9598,#9600,#5914,.T.);
#11805=EDGE_CURVE('',#9588,#9601,#5094,.T.);
#11806=EDGE_CURVE('',#9600,#9589,#5095,.T.);
#11807=EDGE_CURVE('',#9599,#9602,#5915,.T.);
#11808=EDGE_CURVE('',#9603,#9602,#5096,.T.);
#11809=EDGE_CURVE('',#9597,#9603,#5916,.T.);
#11810=EDGE_CURVE('',#9601,#9604,#5917,.T.);
#11811=EDGE_CURVE('',#9602,#9604,#5918,.T.);
#11812=EDGE_CURVE('',#9605,#9588,#5919,.T.);
#11813=EDGE_CURVE('',#9604,#9605,#5097,.T.);
#11814=EDGE_CURVE('',#9587,#9606,#5920,.T.);
#11815=EDGE_CURVE('',#9605,#9606,#5921,.T.);
#11816=EDGE_CURVE('',#9607,#9607,#5098,.T.);
#11817=EDGE_CURVE('',#9608,#9608,#5099,.T.);
#11818=EDGE_CURVE('',#9609,#9609,#5100,.T.);
#11819=EDGE_CURVE('',#9610,#9610,#5101,.T.);
#11820=EDGE_CURVE('',#9611,#9611,#5102,.T.);
#11821=EDGE_CURVE('',#9612,#9612,#5103,.T.);
#11822=EDGE_CURVE('',#9613,#9613,#5104,.T.);
#11823=EDGE_CURVE('',#9581,#9605,#5922,.T.);
#11824=EDGE_CURVE('',#9606,#9582,#5923,.T.);
#11825=EDGE_CURVE('',#9583,#9604,#5924,.T.);
#11826=EDGE_CURVE('',#9584,#9602,#5925,.T.);
#11827=EDGE_CURVE('',#9585,#9603,#5926,.T.);
#11828=EDGE_CURVE('',#9614,#9615,#5927,.T.);
#11829=EDGE_CURVE('',#9615,#9603,#5928,.T.);
#11830=EDGE_CURVE('',#9585,#9614,#5929,.T.);
#11831=EDGE_CURVE('',#9616,#9617,#5930,.T.);
#11832=EDGE_CURVE('',#9617,#9615,#5105,.T.);
#11833=EDGE_CURVE('',#9614,#9616,#5106,.T.);
#11834=EDGE_CURVE('',#9618,#9619,#5931,.T.);
#11835=EDGE_CURVE('',#9619,#9617,#5932,.T.);
#11836=EDGE_CURVE('',#9616,#9618,#5933,.T.);
#11837=EDGE_CURVE('',#9606,#9619,#5107,.T.);
#11838=EDGE_CURVE('',#9618,#9582,#5108,.T.);
#11839=EDGE_CURVE('',#9595,#9615,#5934,.T.);
#11840=EDGE_CURVE('',#9593,#9617,#5935,.T.);
#11841=EDGE_CURVE('',#9591,#9619,#5936,.T.);
#11842=EDGE_CURVE('',#9563,#9620,#5937,.T.);
#11843=EDGE_CURVE('',#9620,#9621,#5109,.T.);
#11844=EDGE_CURVE('',#9621,#9620,#5110,.T.);
#11845=EDGE_CURVE('',#9622,#9622,#5111,.T.);
#11846=EDGE_CURVE('',#9622,#9621,#5938,.T.);
#11847=EDGE_CURVE('',#9569,#9623,#5939,.T.);
#11848=EDGE_CURVE('',#9623,#9624,#5112,.T.);
#11849=EDGE_CURVE('',#9624,#9623,#5113,.T.);
#11850=EDGE_CURVE('',#9625,#9625,#5114,.T.);
#11851=EDGE_CURVE('',#9625,#9624,#5940,.T.);
#11852=EDGE_CURVE('',#9564,#9626,#5941,.T.);
#11853=EDGE_CURVE('',#9626,#9627,#5115,.T.);
#11854=EDGE_CURVE('',#9627,#9626,#5116,.T.);
#11855=EDGE_CURVE('',#9628,#9628,#5117,.T.);
#11856=EDGE_CURVE('',#9628,#9627,#5942,.T.);
#11857=EDGE_CURVE('',#9568,#9629,#5943,.T.);
#11858=EDGE_CURVE('',#9629,#9630,#5118,.T.);
#11859=EDGE_CURVE('',#9630,#9629,#5119,.T.);
#11860=EDGE_CURVE('',#9631,#9631,#5120,.T.);
#11861=EDGE_CURVE('',#9631,#9630,#5944,.T.);
#11862=EDGE_CURVE('',#9607,#9632,#5945,.T.);
#11863=EDGE_CURVE('',#9632,#9633,#5121,.T.);
#11864=EDGE_CURVE('',#9633,#9632,#5122,.T.);
#11865=EDGE_CURVE('',#9634,#9634,#5123,.T.);
#11866=EDGE_CURVE('',#9634,#9633,#5946,.T.);
#11867=EDGE_CURVE('',#9613,#9635,#5947,.T.);
#11868=EDGE_CURVE('',#9635,#9636,#5124,.T.);
#11869=EDGE_CURVE('',#9636,#9635,#5125,.T.);
#11870=EDGE_CURVE('',#9637,#9637,#5126,.T.);
#11871=EDGE_CURVE('',#9637,#9636,#5948,.T.);
#11872=EDGE_CURVE('',#9608,#9638,#5949,.T.);
#11873=EDGE_CURVE('',#9638,#9639,#5127,.T.);
#11874=EDGE_CURVE('',#9639,#9638,#5128,.T.);
#11875=EDGE_CURVE('',#9640,#9640,#5129,.T.);
#11876=EDGE_CURVE('',#9640,#9639,#5950,.T.);
#11877=EDGE_CURVE('',#9567,#9641,#5951,.T.);
#11878=EDGE_CURVE('',#9641,#9641,#5130,.T.);
#11879=EDGE_CURVE('',#9641,#9642,#5952,.T.);
#11880=EDGE_CURVE('',#9642,#9642,#5131,.T.);
#11881=EDGE_CURVE('',#9642,#9643,#5953,.T.);
#11882=EDGE_CURVE('',#9643,#9643,#5132,.T.);
#11883=EDGE_CURVE('',#9566,#9644,#5954,.T.);
#11884=EDGE_CURVE('',#9644,#9644,#5133,.T.);
#11885=EDGE_CURVE('',#9644,#9645,#5955,.T.);
#11886=EDGE_CURVE('',#9645,#9645,#5134,.T.);
#11887=EDGE_CURVE('',#9645,#9646,#5956,.T.);
#11888=EDGE_CURVE('',#9646,#9646,#5135,.T.);
#11889=EDGE_CURVE('',#9565,#9647,#5957,.T.);
#11890=EDGE_CURVE('',#9647,#9647,#5136,.T.);
#11891=EDGE_CURVE('',#9647,#9648,#5958,.T.);
#11892=EDGE_CURVE('',#9648,#9648,#5137,.T.);
#11893=EDGE_CURVE('',#9648,#9649,#5959,.T.);
#11894=EDGE_CURVE('',#9649,#9649,#5138,.T.);
#11895=EDGE_CURVE('',#9609,#9650,#5960,.T.);
#11896=EDGE_CURVE('',#9650,#9650,#5139,.T.);
#11897=EDGE_CURVE('',#9650,#9651,#5961,.T.);
#11898=EDGE_CURVE('',#9651,#9651,#5140,.T.);
#11899=EDGE_CURVE('',#9651,#9652,#5962,.T.);
#11900=EDGE_CURVE('',#9652,#9652,#5141,.T.);
#11901=EDGE_CURVE('',#9610,#9653,#5963,.T.);
#11902=EDGE_CURVE('',#9653,#9653,#5142,.T.);
#11903=EDGE_CURVE('',#9653,#9654,#5964,.T.);
#11904=EDGE_CURVE('',#9654,#9654,#5143,.T.);
#11905=EDGE_CURVE('',#9654,#9655,#5965,.T.);
#11906=EDGE_CURVE('',#9655,#9655,#5144,.T.);
#11907=EDGE_CURVE('',#9611,#9656,#5966,.T.);
#11908=EDGE_CURVE('',#9656,#9656,#5145,.T.);
#11909=EDGE_CURVE('',#9656,#9657,#5967,.T.);
#11910=EDGE_CURVE('',#9657,#9657,#5146,.T.);
#11911=EDGE_CURVE('',#9657,#9658,#5968,.T.);
#11912=EDGE_CURVE('',#9658,#9658,#5147,.T.);
#11913=EDGE_CURVE('',#9612,#9659,#5969,.T.);
#11914=EDGE_CURVE('',#9659,#9659,#5148,.T.);
#11915=EDGE_CURVE('',#9659,#9660,#5970,.T.);
#11916=EDGE_CURVE('',#9660,#9660,#5149,.T.);
#11917=EDGE_CURVE('',#9660,#9661,#5971,.T.);
#11918=EDGE_CURVE('',#9661,#9661,#5150,.T.);
#11919=EDGE_CURVE('',#9614,#9579,#5972,.T.);
#11920=EDGE_CURVE('',#9618,#9575,#5973,.T.);
#11921=EDGE_CURVE('',#9577,#9616,#5974,.T.);
#15067=ORIENTED_EDGE('',*,*,#11711,.T.);
#15068=ORIENTED_EDGE('',*,*,#11712,.T.);
#15069=ORIENTED_EDGE('',*,*,#11713,.T.);
#15070=ORIENTED_EDGE('',*,*,#11714,.T.);
#15071=ORIENTED_EDGE('',*,*,#11715,.T.);
#15072=ORIENTED_EDGE('',*,*,#11716,.T.);
#15073=ORIENTED_EDGE('',*,*,#11711,.F.);
#15074=ORIENTED_EDGE('',*,*,#11717,.T.);
#15075=ORIENTED_EDGE('',*,*,#11718,.T.);
#15076=ORIENTED_EDGE('',*,*,#11719,.T.);
#15077=ORIENTED_EDGE('',*,*,#11715,.F.);
#15078=ORIENTED_EDGE('',*,*,#11720,.T.);
#15079=ORIENTED_EDGE('',*,*,#11721,.T.);
#15080=ORIENTED_EDGE('',*,*,#11722,.T.);
#15081=ORIENTED_EDGE('',*,*,#11718,.F.);
#15082=ORIENTED_EDGE('',*,*,#11723,.T.);
#15083=ORIENTED_EDGE('',*,*,#11724,.T.);
#15084=ORIENTED_EDGE('',*,*,#11725,.T.);
#15085=ORIENTED_EDGE('',*,*,#11721,.F.);
#15086=ORIENTED_EDGE('',*,*,#11726,.T.);
#15087=ORIENTED_EDGE('',*,*,#11727,.T.);
#15088=ORIENTED_EDGE('',*,*,#11728,.T.);
#15089=ORIENTED_EDGE('',*,*,#11724,.F.);
#15090=ORIENTED_EDGE('',*,*,#11729,.T.);
#15091=ORIENTED_EDGE('',*,*,#11730,.T.);
#15092=ORIENTED_EDGE('',*,*,#11731,.T.);
#15093=ORIENTED_EDGE('',*,*,#11727,.F.);
#15094=ORIENTED_EDGE('',*,*,#11732,.T.);
#15095=ORIENTED_EDGE('',*,*,#11713,.F.);
#15096=ORIENTED_EDGE('',*,*,#11733,.T.);
#15097=ORIENTED_EDGE('',*,*,#11730,.F.);
#15098=ORIENTED_EDGE('',*,*,#11734,.T.);
#15099=ORIENTED_EDGE('',*,*,#11728,.F.);
#15100=ORIENTED_EDGE('',*,*,#11735,.T.);
#15101=ORIENTED_EDGE('',*,*,#11736,.F.);
#15102=ORIENTED_EDGE('',*,*,#11737,.F.);
#15103=ORIENTED_EDGE('',*,*,#11731,.F.);
#15104=ORIENTED_EDGE('',*,*,#11738,.T.);
#15105=ORIENTED_EDGE('',*,*,#11739,.F.);
#15106=ORIENTED_EDGE('',*,*,#11735,.F.);
#15107=ORIENTED_EDGE('',*,*,#11733,.F.);
#15108=ORIENTED_EDGE('',*,*,#11740,.F.);
#15109=ORIENTED_EDGE('',*,*,#11741,.F.);
#15110=ORIENTED_EDGE('',*,*,#11738,.F.);
#15111=ORIENTED_EDGE('',*,*,#11712,.F.);
#15112=ORIENTED_EDGE('',*,*,#11742,.T.);
#15113=ORIENTED_EDGE('',*,*,#11743,.F.);
#15114=ORIENTED_EDGE('',*,*,#11740,.T.);
#15115=ORIENTED_EDGE('',*,*,#11714,.F.);
#15116=ORIENTED_EDGE('',*,*,#11734,.F.);
#15117=ORIENTED_EDGE('',*,*,#11732,.F.);
#15118=ORIENTED_EDGE('',*,*,#11729,.F.);
#15119=ORIENTED_EDGE('',*,*,#11726,.F.);
#15120=ORIENTED_EDGE('',*,*,#11723,.F.);
#15121=ORIENTED_EDGE('',*,*,#11720,.F.);
#15122=ORIENTED_EDGE('',*,*,#11717,.F.);
#15123=ORIENTED_EDGE('',*,*,#11744,.F.);
#15124=ORIENTED_EDGE('',*,*,#11745,.F.);
#15125=ORIENTED_EDGE('',*,*,#11746,.T.);
#15126=ORIENTED_EDGE('',*,*,#11747,.T.);
#15127=ORIENTED_EDGE('',*,*,#11748,.T.);
#15128=ORIENTED_EDGE('',*,*,#11749,.F.);
#15129=ORIENTED_EDGE('',*,*,#11750,.F.);
#15130=ORIENTED_EDGE('',*,*,#11751,.T.);
#15131=ORIENTED_EDGE('',*,*,#11743,.T.);
#15132=ORIENTED_EDGE('',*,*,#11752,.T.);
#15133=ORIENTED_EDGE('',*,*,#11753,.T.);
#15134=ORIENTED_EDGE('',*,*,#11754,.T.);
#15135=ORIENTED_EDGE('',*,*,#11741,.T.);
#15136=ORIENTED_EDGE('',*,*,#11751,.F.);
#15137=ORIENTED_EDGE('',*,*,#11755,.T.);
#15138=ORIENTED_EDGE('',*,*,#11756,.T.);
#15139=ORIENTED_EDGE('',*,*,#11739,.T.);
#15140=ORIENTED_EDGE('',*,*,#11754,.F.);
#15141=ORIENTED_EDGE('',*,*,#11757,.T.);
#15142=ORIENTED_EDGE('',*,*,#11758,.T.);
#15143=ORIENTED_EDGE('',*,*,#11736,.T.);
#15144=ORIENTED_EDGE('',*,*,#11756,.F.);
#15145=ORIENTED_EDGE('',*,*,#11759,.T.);
#15146=ORIENTED_EDGE('',*,*,#11760,.T.);
#15147=ORIENTED_EDGE('',*,*,#11761,.T.);
#15148=ORIENTED_EDGE('',*,*,#11758,.F.);
#15149=ORIENTED_EDGE('',*,*,#11762,.T.);
#15150=ORIENTED_EDGE('',*,*,#11763,.T.);
#15151=ORIENTED_EDGE('',*,*,#11764,.T.);
#15152=ORIENTED_EDGE('',*,*,#11760,.F.);
#15153=ORIENTED_EDGE('',*,*,#11765,.T.);
#15154=ORIENTED_EDGE('',*,*,#11766,.T.);
#15155=ORIENTED_EDGE('',*,*,#11767,.T.);
#15156=ORIENTED_EDGE('',*,*,#11763,.F.);
#15157=ORIENTED_EDGE('',*,*,#11768,.T.);
#15158=ORIENTED_EDGE('',*,*,#11752,.F.);
#15159=ORIENTED_EDGE('',*,*,#11769,.T.);
#15160=ORIENTED_EDGE('',*,*,#11766,.F.);
#15161=ORIENTED_EDGE('',*,*,#11770,.T.);
#15162=ORIENTED_EDGE('',*,*,#11759,.F.);
#15163=ORIENTED_EDGE('',*,*,#11771,.F.);
#15164=ORIENTED_EDGE('',*,*,#11772,.F.);
#15165=ORIENTED_EDGE('',*,*,#11773,.F.);
#15166=ORIENTED_EDGE('',*,*,#11757,.F.);
#15167=ORIENTED_EDGE('',*,*,#11774,.T.);
#15168=ORIENTED_EDGE('',*,*,#11775,.F.);
#15169=ORIENTED_EDGE('',*,*,#11771,.T.);
#15170=ORIENTED_EDGE('',*,*,#11755,.F.);
#15171=ORIENTED_EDGE('',*,*,#11776,.F.);
#15172=ORIENTED_EDGE('',*,*,#11777,.F.);
#15173=ORIENTED_EDGE('',*,*,#11774,.F.);
#15174=ORIENTED_EDGE('',*,*,#11753,.F.);
#15175=ORIENTED_EDGE('',*,*,#11778,.T.);
#15176=ORIENTED_EDGE('',*,*,#11779,.F.);
#15177=ORIENTED_EDGE('',*,*,#11776,.T.);
#15178=ORIENTED_EDGE('',*,*,#11722,.F.);
#15179=ORIENTED_EDGE('',*,*,#11780,.T.);
#15180=ORIENTED_EDGE('',*,*,#11764,.F.);
#15181=ORIENTED_EDGE('',*,*,#11781,.F.);
#15182=ORIENTED_EDGE('',*,*,#11719,.F.);
#15183=ORIENTED_EDGE('',*,*,#11781,.T.);
#15184=ORIENTED_EDGE('',*,*,#11767,.F.);
#15185=ORIENTED_EDGE('',*,*,#11782,.F.);
#15186=ORIENTED_EDGE('',*,*,#11716,.F.);
#15187=ORIENTED_EDGE('',*,*,#11782,.T.);
#15188=ORIENTED_EDGE('',*,*,#11769,.F.);
#15189=ORIENTED_EDGE('',*,*,#11742,.F.);
#15190=ORIENTED_EDGE('',*,*,#11783,.T.);
#15191=ORIENTED_EDGE('',*,*,#11784,.T.);
#15192=ORIENTED_EDGE('',*,*,#11785,.T.);
#15193=ORIENTED_EDGE('',*,*,#11786,.T.);
#15194=ORIENTED_EDGE('',*,*,#11787,.T.);
#15195=ORIENTED_EDGE('',*,*,#11788,.T.);
#15196=ORIENTED_EDGE('',*,*,#11783,.F.);
#15197=ORIENTED_EDGE('',*,*,#11789,.T.);
#15198=ORIENTED_EDGE('',*,*,#11790,.T.);
#15199=ORIENTED_EDGE('',*,*,#11791,.T.);
#15200=ORIENTED_EDGE('',*,*,#11787,.F.);
#15201=ORIENTED_EDGE('',*,*,#11792,.T.);
#15202=ORIENTED_EDGE('',*,*,#11793,.T.);
#15203=ORIENTED_EDGE('',*,*,#11794,.T.);
#15204=ORIENTED_EDGE('',*,*,#11790,.F.);
#15205=ORIENTED_EDGE('',*,*,#11795,.T.);
#15206=ORIENTED_EDGE('',*,*,#11796,.T.);
#15207=ORIENTED_EDGE('',*,*,#11797,.T.);
#15208=ORIENTED_EDGE('',*,*,#11793,.F.);
#15209=ORIENTED_EDGE('',*,*,#11798,.T.);
#15210=ORIENTED_EDGE('',*,*,#11799,.T.);
#15211=ORIENTED_EDGE('',*,*,#11800,.T.);
#15212=ORIENTED_EDGE('',*,*,#11796,.F.);
#15213=ORIENTED_EDGE('',*,*,#11801,.T.);
#15214=ORIENTED_EDGE('',*,*,#11802,.T.);
#15215=ORIENTED_EDGE('',*,*,#11803,.T.);
#15216=ORIENTED_EDGE('',*,*,#11799,.F.);
#15217=ORIENTED_EDGE('',*,*,#11804,.T.);
#15218=ORIENTED_EDGE('',*,*,#11785,.F.);
#15219=ORIENTED_EDGE('',*,*,#11805,.T.);
#15220=ORIENTED_EDGE('',*,*,#11802,.F.);
#15221=ORIENTED_EDGE('',*,*,#11806,.T.);
#15222=ORIENTED_EDGE('',*,*,#11800,.F.);
#15223=ORIENTED_EDGE('',*,*,#11807,.T.);
#15224=ORIENTED_EDGE('',*,*,#11808,.F.);
#15225=ORIENTED_EDGE('',*,*,#11809,.F.);
#15226=ORIENTED_EDGE('',*,*,#11803,.F.);
#15227=ORIENTED_EDGE('',*,*,#11810,.T.);
#15228=ORIENTED_EDGE('',*,*,#11811,.F.);
#15229=ORIENTED_EDGE('',*,*,#11807,.F.);
#15230=ORIENTED_EDGE('',*,*,#11805,.F.);
#15231=ORIENTED_EDGE('',*,*,#11812,.F.);
#15232=ORIENTED_EDGE('',*,*,#11813,.F.);
#15233=ORIENTED_EDGE('',*,*,#11810,.F.);
#15234=ORIENTED_EDGE('',*,*,#11784,.F.);
#15235=ORIENTED_EDGE('',*,*,#11814,.T.);
#15236=ORIENTED_EDGE('',*,*,#11815,.F.);
#15237=ORIENTED_EDGE('',*,*,#11812,.T.);
#15238=ORIENTED_EDGE('',*,*,#11786,.F.);
#15239=ORIENTED_EDGE('',*,*,#11806,.F.);
#15240=ORIENTED_EDGE('',*,*,#11804,.F.);
#15241=ORIENTED_EDGE('',*,*,#11801,.F.);
#15242=ORIENTED_EDGE('',*,*,#11798,.F.);
#15243=ORIENTED_EDGE('',*,*,#11795,.F.);
#15244=ORIENTED_EDGE('',*,*,#11792,.F.);
#15245=ORIENTED_EDGE('',*,*,#11789,.F.);
#15246=ORIENTED_EDGE('',*,*,#11816,.F.);
#15247=ORIENTED_EDGE('',*,*,#11817,.F.);
#15248=ORIENTED_EDGE('',*,*,#11818,.T.);
#15249=ORIENTED_EDGE('',*,*,#11819,.T.);
#15250=ORIENTED_EDGE('',*,*,#11820,.T.);
#15251=ORIENTED_EDGE('',*,*,#11821,.T.);
#15252=ORIENTED_EDGE('',*,*,#11822,.F.);
#15253=ORIENTED_EDGE('',*,*,#11823,.T.);
#15254=ORIENTED_EDGE('',*,*,#11815,.T.);
#15255=ORIENTED_EDGE('',*,*,#11824,.T.);
#15256=ORIENTED_EDGE('',*,*,#11772,.T.);
#15257=ORIENTED_EDGE('',*,*,#11825,.T.);
#15258=ORIENTED_EDGE('',*,*,#11813,.T.);
#15259=ORIENTED_EDGE('',*,*,#11823,.F.);
#15260=ORIENTED_EDGE('',*,*,#11775,.T.);
#15261=ORIENTED_EDGE('',*,*,#11826,.T.);
#15262=ORIENTED_EDGE('',*,*,#11811,.T.);
#15263=ORIENTED_EDGE('',*,*,#11825,.F.);
#15264=ORIENTED_EDGE('',*,*,#11777,.T.);
#15265=ORIENTED_EDGE('',*,*,#11827,.T.);
#15266=ORIENTED_EDGE('',*,*,#11808,.T.);
#15267=ORIENTED_EDGE('',*,*,#11826,.F.);
#15268=ORIENTED_EDGE('',*,*,#11779,.T.);
#15269=ORIENTED_EDGE('',*,*,#11828,.T.);
#15270=ORIENTED_EDGE('',*,*,#11829,.T.);
#15271=ORIENTED_EDGE('',*,*,#11827,.F.);
#15272=ORIENTED_EDGE('',*,*,#11830,.T.);
#15273=ORIENTED_EDGE('',*,*,#11831,.T.);
#15274=ORIENTED_EDGE('',*,*,#11832,.T.);
#15275=ORIENTED_EDGE('',*,*,#11828,.F.);
#15276=ORIENTED_EDGE('',*,*,#11833,.T.);
#15277=ORIENTED_EDGE('',*,*,#11834,.T.);
#15278=ORIENTED_EDGE('',*,*,#11835,.T.);
#15279=ORIENTED_EDGE('',*,*,#11831,.F.);
#15280=ORIENTED_EDGE('',*,*,#11836,.T.);
#15281=ORIENTED_EDGE('',*,*,#11824,.F.);
#15282=ORIENTED_EDGE('',*,*,#11837,.T.);
#15283=ORIENTED_EDGE('',*,*,#11834,.F.);
#15284=ORIENTED_EDGE('',*,*,#11838,.T.);
#15285=ORIENTED_EDGE('',*,*,#11794,.F.);
#15286=ORIENTED_EDGE('',*,*,#11839,.T.);
#15287=ORIENTED_EDGE('',*,*,#11832,.F.);
#15288=ORIENTED_EDGE('',*,*,#11840,.F.);
#15289=ORIENTED_EDGE('',*,*,#11791,.F.);
#15290=ORIENTED_EDGE('',*,*,#11840,.T.);
#15291=ORIENTED_EDGE('',*,*,#11835,.F.);
#15292=ORIENTED_EDGE('',*,*,#11841,.F.);
#15293=ORIENTED_EDGE('',*,*,#11788,.F.);
#15294=ORIENTED_EDGE('',*,*,#11841,.T.);
#15295=ORIENTED_EDGE('',*,*,#11837,.F.);
#15296=ORIENTED_EDGE('',*,*,#11814,.F.);
#15297=ORIENTED_EDGE('',*,*,#11744,.T.);
#15298=ORIENTED_EDGE('',*,*,#11842,.T.);
#15299=ORIENTED_EDGE('',*,*,#11843,.T.);
#15300=ORIENTED_EDGE('',*,*,#11844,.T.);
#15301=ORIENTED_EDGE('',*,*,#11842,.F.);
#15302=ORIENTED_EDGE('',*,*,#11845,.F.);
#15303=ORIENTED_EDGE('',*,*,#11846,.T.);
#15304=ORIENTED_EDGE('',*,*,#11843,.F.);
#15305=ORIENTED_EDGE('',*,*,#11844,.F.);
#15306=ORIENTED_EDGE('',*,*,#11846,.F.);
#15307=ORIENTED_EDGE('',*,*,#11750,.T.);
#15308=ORIENTED_EDGE('',*,*,#11847,.T.);
#15309=ORIENTED_EDGE('',*,*,#11848,.T.);
#15310=ORIENTED_EDGE('',*,*,#11849,.T.);
#15311=ORIENTED_EDGE('',*,*,#11847,.F.);
#15312=ORIENTED_EDGE('',*,*,#11850,.F.);
#15313=ORIENTED_EDGE('',*,*,#11851,.T.);
#15314=ORIENTED_EDGE('',*,*,#11848,.F.);
#15315=ORIENTED_EDGE('',*,*,#11849,.F.);
#15316=ORIENTED_EDGE('',*,*,#11851,.F.);
#15317=ORIENTED_EDGE('',*,*,#11745,.T.);
#15318=ORIENTED_EDGE('',*,*,#11852,.T.);
#15319=ORIENTED_EDGE('',*,*,#11853,.T.);
#15320=ORIENTED_EDGE('',*,*,#11854,.T.);
#15321=ORIENTED_EDGE('',*,*,#11852,.F.);
#15322=ORIENTED_EDGE('',*,*,#11855,.F.);
#15323=ORIENTED_EDGE('',*,*,#11856,.T.);
#15324=ORIENTED_EDGE('',*,*,#11853,.F.);
#15325=ORIENTED_EDGE('',*,*,#11854,.F.);
#15326=ORIENTED_EDGE('',*,*,#11856,.F.);
#15327=ORIENTED_EDGE('',*,*,#11749,.T.);
#15328=ORIENTED_EDGE('',*,*,#11857,.T.);
#15329=ORIENTED_EDGE('',*,*,#11858,.T.);
#15330=ORIENTED_EDGE('',*,*,#11859,.T.);
#15331=ORIENTED_EDGE('',*,*,#11857,.F.);
#15332=ORIENTED_EDGE('',*,*,#11860,.F.);
#15333=ORIENTED_EDGE('',*,*,#11861,.T.);
#15334=ORIENTED_EDGE('',*,*,#11858,.F.);
#15335=ORIENTED_EDGE('',*,*,#11859,.F.);
#15336=ORIENTED_EDGE('',*,*,#11861,.F.);
#15337=ORIENTED_EDGE('',*,*,#11816,.T.);
#15338=ORIENTED_EDGE('',*,*,#11862,.T.);
#15339=ORIENTED_EDGE('',*,*,#11863,.T.);
#15340=ORIENTED_EDGE('',*,*,#11864,.T.);
#15341=ORIENTED_EDGE('',*,*,#11862,.F.);
#15342=ORIENTED_EDGE('',*,*,#11865,.F.);
#15343=ORIENTED_EDGE('',*,*,#11866,.T.);
#15344=ORIENTED_EDGE('',*,*,#11863,.F.);
#15345=ORIENTED_EDGE('',*,*,#11864,.F.);
#15346=ORIENTED_EDGE('',*,*,#11866,.F.);
#15347=ORIENTED_EDGE('',*,*,#11822,.T.);
#15348=ORIENTED_EDGE('',*,*,#11867,.T.);
#15349=ORIENTED_EDGE('',*,*,#11868,.T.);
#15350=ORIENTED_EDGE('',*,*,#11869,.T.);
#15351=ORIENTED_EDGE('',*,*,#11867,.F.);
#15352=ORIENTED_EDGE('',*,*,#11870,.F.);
#15353=ORIENTED_EDGE('',*,*,#11871,.T.);
#15354=ORIENTED_EDGE('',*,*,#11868,.F.);
#15355=ORIENTED_EDGE('',*,*,#11869,.F.);
#15356=ORIENTED_EDGE('',*,*,#11871,.F.);
#15357=ORIENTED_EDGE('',*,*,#11817,.T.);
#15358=ORIENTED_EDGE('',*,*,#11872,.T.);
#15359=ORIENTED_EDGE('',*,*,#11873,.T.);
#15360=ORIENTED_EDGE('',*,*,#11874,.T.);
#15361=ORIENTED_EDGE('',*,*,#11872,.F.);
#15362=ORIENTED_EDGE('',*,*,#11875,.F.);
#15363=ORIENTED_EDGE('',*,*,#11876,.T.);
#15364=ORIENTED_EDGE('',*,*,#11873,.F.);
#15365=ORIENTED_EDGE('',*,*,#11874,.F.);
#15366=ORIENTED_EDGE('',*,*,#11876,.F.);
#15367=ORIENTED_EDGE('',*,*,#11748,.F.);
#15368=ORIENTED_EDGE('',*,*,#11877,.T.);
#15369=ORIENTED_EDGE('',*,*,#11878,.T.);
#15370=ORIENTED_EDGE('',*,*,#11877,.F.);
#15371=ORIENTED_EDGE('',*,*,#11878,.F.);
#15372=ORIENTED_EDGE('',*,*,#11879,.T.);
#15373=ORIENTED_EDGE('',*,*,#11880,.T.);
#15374=ORIENTED_EDGE('',*,*,#11879,.F.);
#15375=ORIENTED_EDGE('',*,*,#11880,.F.);
#15376=ORIENTED_EDGE('',*,*,#11881,.T.);
#15377=ORIENTED_EDGE('',*,*,#11882,.T.);
#15378=ORIENTED_EDGE('',*,*,#11881,.F.);
#15379=ORIENTED_EDGE('',*,*,#11875,.T.);
#15380=ORIENTED_EDGE('',*,*,#11882,.F.);
#15381=ORIENTED_EDGE('',*,*,#11747,.F.);
#15382=ORIENTED_EDGE('',*,*,#11883,.T.);
#15383=ORIENTED_EDGE('',*,*,#11884,.T.);
#15384=ORIENTED_EDGE('',*,*,#11883,.F.);
#15385=ORIENTED_EDGE('',*,*,#11884,.F.);
#15386=ORIENTED_EDGE('',*,*,#11885,.T.);
#15387=ORIENTED_EDGE('',*,*,#11886,.T.);
#15388=ORIENTED_EDGE('',*,*,#11885,.F.);
#15389=ORIENTED_EDGE('',*,*,#11886,.F.);
#15390=ORIENTED_EDGE('',*,*,#11887,.T.);
#15391=ORIENTED_EDGE('',*,*,#11888,.T.);
#15392=ORIENTED_EDGE('',*,*,#11887,.F.);
#15393=ORIENTED_EDGE('',*,*,#11870,.T.);
#15394=ORIENTED_EDGE('',*,*,#11888,.F.);
#15395=ORIENTED_EDGE('',*,*,#11746,.F.);
#15396=ORIENTED_EDGE('',*,*,#11889,.T.);
#15397=ORIENTED_EDGE('',*,*,#11890,.T.);
#15398=ORIENTED_EDGE('',*,*,#11889,.F.);
#15399=ORIENTED_EDGE('',*,*,#11890,.F.);
#15400=ORIENTED_EDGE('',*,*,#11891,.T.);
#15401=ORIENTED_EDGE('',*,*,#11892,.T.);
#15402=ORIENTED_EDGE('',*,*,#11891,.F.);
#15403=ORIENTED_EDGE('',*,*,#11892,.F.);
#15404=ORIENTED_EDGE('',*,*,#11893,.T.);
#15405=ORIENTED_EDGE('',*,*,#11894,.T.);
#15406=ORIENTED_EDGE('',*,*,#11893,.F.);
#15407=ORIENTED_EDGE('',*,*,#11865,.T.);
#15408=ORIENTED_EDGE('',*,*,#11894,.F.);
#15409=ORIENTED_EDGE('',*,*,#11818,.F.);
#15410=ORIENTED_EDGE('',*,*,#11895,.T.);
#15411=ORIENTED_EDGE('',*,*,#11896,.T.);
#15412=ORIENTED_EDGE('',*,*,#11895,.F.);
#15413=ORIENTED_EDGE('',*,*,#11896,.F.);
#15414=ORIENTED_EDGE('',*,*,#11897,.T.);
#15415=ORIENTED_EDGE('',*,*,#11898,.T.);
#15416=ORIENTED_EDGE('',*,*,#11897,.F.);
#15417=ORIENTED_EDGE('',*,*,#11898,.F.);
#15418=ORIENTED_EDGE('',*,*,#11899,.T.);
#15419=ORIENTED_EDGE('',*,*,#11900,.T.);
#15420=ORIENTED_EDGE('',*,*,#11899,.F.);
#15421=ORIENTED_EDGE('',*,*,#11860,.T.);
#15422=ORIENTED_EDGE('',*,*,#11900,.F.);
#15423=ORIENTED_EDGE('',*,*,#11819,.F.);
#15424=ORIENTED_EDGE('',*,*,#11901,.T.);
#15425=ORIENTED_EDGE('',*,*,#11902,.T.);
#15426=ORIENTED_EDGE('',*,*,#11901,.F.);
#15427=ORIENTED_EDGE('',*,*,#11902,.F.);
#15428=ORIENTED_EDGE('',*,*,#11903,.T.);
#15429=ORIENTED_EDGE('',*,*,#11904,.T.);
#15430=ORIENTED_EDGE('',*,*,#11903,.F.);
#15431=ORIENTED_EDGE('',*,*,#11904,.F.);
#15432=ORIENTED_EDGE('',*,*,#11905,.T.);
#15433=ORIENTED_EDGE('',*,*,#11906,.T.);
#15434=ORIENTED_EDGE('',*,*,#11905,.F.);
#15435=ORIENTED_EDGE('',*,*,#11855,.T.);
#15436=ORIENTED_EDGE('',*,*,#11906,.F.);
#15437=ORIENTED_EDGE('',*,*,#11820,.F.);
#15438=ORIENTED_EDGE('',*,*,#11907,.T.);
#15439=ORIENTED_EDGE('',*,*,#11908,.T.);
#15440=ORIENTED_EDGE('',*,*,#11907,.F.);
#15441=ORIENTED_EDGE('',*,*,#11908,.F.);
#15442=ORIENTED_EDGE('',*,*,#11909,.T.);
#15443=ORIENTED_EDGE('',*,*,#11910,.T.);
#15444=ORIENTED_EDGE('',*,*,#11909,.F.);
#15445=ORIENTED_EDGE('',*,*,#11910,.F.);
#15446=ORIENTED_EDGE('',*,*,#11911,.T.);
#15447=ORIENTED_EDGE('',*,*,#11912,.T.);
#15448=ORIENTED_EDGE('',*,*,#11911,.F.);
#15449=ORIENTED_EDGE('',*,*,#11850,.T.);
#15450=ORIENTED_EDGE('',*,*,#11912,.F.);
#15451=ORIENTED_EDGE('',*,*,#11821,.F.);
#15452=ORIENTED_EDGE('',*,*,#11913,.T.);
#15453=ORIENTED_EDGE('',*,*,#11914,.T.);
#15454=ORIENTED_EDGE('',*,*,#11913,.F.);
#15455=ORIENTED_EDGE('',*,*,#11914,.F.);
#15456=ORIENTED_EDGE('',*,*,#11915,.T.);
#15457=ORIENTED_EDGE('',*,*,#11916,.T.);
#15458=ORIENTED_EDGE('',*,*,#11915,.F.);
#15459=ORIENTED_EDGE('',*,*,#11916,.F.);
#15460=ORIENTED_EDGE('',*,*,#11917,.T.);
#15461=ORIENTED_EDGE('',*,*,#11918,.T.);
#15462=ORIENTED_EDGE('',*,*,#11917,.F.);
#15463=ORIENTED_EDGE('',*,*,#11845,.T.);
#15464=ORIENTED_EDGE('',*,*,#11918,.F.);
#15465=ORIENTED_EDGE('',*,*,#11797,.F.);
#15466=ORIENTED_EDGE('',*,*,#11809,.T.);
#15467=ORIENTED_EDGE('',*,*,#11829,.F.);
#15468=ORIENTED_EDGE('',*,*,#11839,.F.);
#15469=ORIENTED_EDGE('',*,*,#11725,.F.);
#15470=ORIENTED_EDGE('',*,*,#11737,.T.);
#15471=ORIENTED_EDGE('',*,*,#11761,.F.);
#15472=ORIENTED_EDGE('',*,*,#11780,.F.);
#15473=ORIENTED_EDGE('',*,*,#11770,.F.);
#15474=ORIENTED_EDGE('',*,*,#11919,.F.);
#15475=ORIENTED_EDGE('',*,*,#11830,.F.);
#15476=ORIENTED_EDGE('',*,*,#11778,.F.);
#15477=ORIENTED_EDGE('',*,*,#11762,.F.);
#15478=ORIENTED_EDGE('',*,*,#11773,.T.);
#15479=ORIENTED_EDGE('',*,*,#11838,.F.);
#15480=ORIENTED_EDGE('',*,*,#11920,.T.);
#15481=ORIENTED_EDGE('',*,*,#11768,.F.);
#15482=ORIENTED_EDGE('',*,*,#11921,.T.);
#15483=ORIENTED_EDGE('',*,*,#11833,.F.);
#15484=ORIENTED_EDGE('',*,*,#11919,.T.);
#15485=ORIENTED_EDGE('',*,*,#11765,.F.);
#15486=ORIENTED_EDGE('',*,*,#11920,.F.);
#15487=ORIENTED_EDGE('',*,*,#11836,.F.);
#15488=ORIENTED_EDGE('',*,*,#11921,.F.);
#21779=CONICAL_SURFACE('',#23498,0.495606601717798,1.17809724509618);
#21780=CONICAL_SURFACE('',#23502,0.495606601717798,1.17809724509618);
#21781=CONICAL_SURFACE('',#23506,0.495606601717798,1.17809724509618);
#21782=CONICAL_SURFACE('',#23510,0.495606601717798,1.17809724509618);
#21783=CONICAL_SURFACE('',#23515,0.55,0.785398163397448);
#21784=CONICAL_SURFACE('',#23518,0.55,0.785398163397448);
#21785=CONICAL_SURFACE('',#23528,0.589393398282202,0.392699081698717);
#21786=CONICAL_SURFACE('',#23531,0.589393398282202,0.392699081698717);
#21787=CONICAL_SURFACE('',#23534,0.589393398282202,0.392699081698717);
#21788=CONICAL_SURFACE('',#23538,0.589393398282202,0.392699081698717);
#21789=CONICAL_SURFACE('',#23549,0.55,0.785398163397448);
#21790=CONICAL_SURFACE('',#23552,0.545606601717798,1.17809724509617);
#21791=CONICAL_SURFACE('',#23556,0.545606601717798,1.17809724509617);
#21792=CONICAL_SURFACE('',#23560,0.545606601717798,1.17809724509617);
#21793=CONICAL_SURFACE('',#23564,0.545606601717798,1.17809724509617);
#21794=CONICAL_SURFACE('',#23567,0.575,0.785398163397449);
#21795=CONICAL_SURFACE('',#23570,0.575,0.785398163397449);
#21796=CONICAL_SURFACE('',#23582,0.589393398282202,0.392699081698719);
#21797=CONICAL_SURFACE('',#23584,0.589393398282202,0.392699081698719);
#21798=CONICAL_SURFACE('',#23586,0.589393398282202,0.392699081698719);
#21799=CONICAL_SURFACE('',#23590,0.589393398282202,0.392699081698719);
#21800=CONICAL_SURFACE('',#23593,0.575,0.785398163397449);
#21801=CONICAL_SURFACE('',#23595,0.575,0.785398163397449);
#21802=CONICAL_SURFACE('',#23596,0.565,0.785398163397452);
#21803=CONICAL_SURFACE('',#23601,0.565,0.785398163397452);
#21804=CONICAL_SURFACE('',#23606,0.565,0.785398163397452);
#21805=CONICAL_SURFACE('',#23611,0.565,0.785398163397452);
#21806=CONICAL_SURFACE('',#23616,0.515,0.785398163397445);
#21807=CONICAL_SURFACE('',#23621,0.515,0.785398163397449);
#21808=CONICAL_SURFACE('',#23626,0.515,0.785398163397452);
#21809=CONICAL_SURFACE('',#23631,0.2875,0.321750554396636);
#21810=CONICAL_SURFACE('',#23635,0.2875,0.785398163397439);
#21811=CONICAL_SURFACE('',#23638,0.2875,0.321750554396642);
#21812=CONICAL_SURFACE('',#23642,0.2875,0.78539816339745);
#21813=CONICAL_SURFACE('',#23645,0.2875,0.321750554396636);
#21814=CONICAL_SURFACE('',#23649,0.2875,0.785398163397439);
#21815=CONICAL_SURFACE('',#23652,0.342499999999999,0.321750554396636);
#21816=CONICAL_SURFACE('',#23656,0.342499999999999,0.785398163397437);
#21817=CONICAL_SURFACE('',#23659,0.342499999999999,0.321750554396636);
#21818=CONICAL_SURFACE('',#23663,0.342499999999999,0.785398163397437);
#21819=CONICAL_SURFACE('',#23666,0.342499999999999,0.321750554396636);
#21820=CONICAL_SURFACE('',#23670,0.342499999999999,0.785398163397437);
#21821=CONICAL_SURFACE('',#23673,0.342499999999999,0.321750554396636);
#21822=CONICAL_SURFACE('',#23677,0.342499999999999,0.785398163397437);
#21823=CONICAL_SURFACE('',#23681,0.55,0.785398163397448);
#21975=ADVANCED_FACE('',(#2236),#21779,.T.);
#21976=ADVANCED_FACE('',(#2237),#1448,.T.);
#21977=ADVANCED_FACE('',(#2238),#21780,.T.);
#21978=ADVANCED_FACE('',(#2239),#1449,.T.);
#21979=ADVANCED_FACE('',(#2240),#21781,.T.);
#21980=ADVANCED_FACE('',(#2241),#1450,.T.);
#21981=ADVANCED_FACE('',(#2242),#21782,.T.);
#21982=ADVANCED_FACE('',(#2243),#1451,.T.);
#21983=ADVANCED_FACE('',(#2244),#1452,.T.);
#21984=ADVANCED_FACE('',(#2245),#21783,.T.);
#21985=ADVANCED_FACE('',(#2246),#1453,.T.);
#21986=ADVANCED_FACE('',(#2247),#21784,.T.);
#21987=ADVANCED_FACE('',(#2248,#1277,#1278,#1279,#1280,#1281,#1282,#1283),
#1454,.T.);
#21988=ADVANCED_FACE('',(#2249),#21785,.T.);
#21989=ADVANCED_FACE('',(#2250),#1455,.T.);
#21990=ADVANCED_FACE('',(#2251),#21786,.T.);
#21991=ADVANCED_FACE('',(#2252),#1456,.T.);
#21992=ADVANCED_FACE('',(#2253),#21787,.T.);
#21993=ADVANCED_FACE('',(#2254),#1457,.T.);
#21994=ADVANCED_FACE('',(#2255),#21788,.T.);
#21995=ADVANCED_FACE('',(#2256),#1458,.T.);
#21996=ADVANCED_FACE('',(#2257),#1459,.T.);
#21997=ADVANCED_FACE('',(#2258),#943,.T.);
#21998=ADVANCED_FACE('',(#2259),#1460,.T.);
#21999=ADVANCED_FACE('',(#2260),#944,.T.);
#22000=ADVANCED_FACE('',(#2261),#1461,.T.);
#22001=ADVANCED_FACE('',(#2262),#21789,.T.);
#22002=ADVANCED_FACE('',(#2263),#1462,.T.);
#22003=ADVANCED_FACE('',(#2264),#1463,.T.);
#22004=ADVANCED_FACE('',(#2265),#21790,.T.);
#22005=ADVANCED_FACE('',(#2266),#1464,.T.);
#22006=ADVANCED_FACE('',(#2267),#21791,.T.);
#22007=ADVANCED_FACE('',(#2268),#1465,.T.);
#22008=ADVANCED_FACE('',(#2269),#21792,.T.);
#22009=ADVANCED_FACE('',(#2270),#1466,.T.);
#22010=ADVANCED_FACE('',(#2271),#21793,.T.);
#22011=ADVANCED_FACE('',(#2272),#21794,.T.);
#22012=ADVANCED_FACE('',(#2273),#1467,.T.);
#22013=ADVANCED_FACE('',(#2274),#21795,.T.);
#22014=ADVANCED_FACE('',(#2275),#1468,.T.);
#22015=ADVANCED_FACE('',(#2276,#1284,#1285,#1286,#1287,#1288,#1289,#1290),
#1469,.F.);
#22016=ADVANCED_FACE('',(#2277),#1470,.T.);
#22017=ADVANCED_FACE('',(#2278),#21796,.T.);
#22018=ADVANCED_FACE('',(#2279),#1471,.T.);
#22019=ADVANCED_FACE('',(#2280),#21797,.T.);
#22020=ADVANCED_FACE('',(#2281),#1472,.T.);
#22021=ADVANCED_FACE('',(#2282),#21798,.T.);
#22022=ADVANCED_FACE('',(#2283),#1473,.T.);
#22023=ADVANCED_FACE('',(#2284),#21799,.T.);
#22024=ADVANCED_FACE('',(#2285),#21800,.T.);
#22025=ADVANCED_FACE('',(#2286),#1474,.T.);
#22026=ADVANCED_FACE('',(#2287),#21801,.T.);
#22027=ADVANCED_FACE('',(#2288),#21802,.F.);
#22028=ADVANCED_FACE('',(#2289),#945,.F.);
#22029=ADVANCED_FACE('',(#2290),#21803,.F.);
#22030=ADVANCED_FACE('',(#2291),#946,.F.);
#22031=ADVANCED_FACE('',(#2292),#21804,.F.);
#22032=ADVANCED_FACE('',(#2293),#947,.F.);
#22033=ADVANCED_FACE('',(#2294),#21805,.F.);
#22034=ADVANCED_FACE('',(#2295),#948,.F.);
#22035=ADVANCED_FACE('',(#2296),#21806,.F.);
#22036=ADVANCED_FACE('',(#2297),#949,.F.);
#22037=ADVANCED_FACE('',(#2298),#21807,.F.);
#22038=ADVANCED_FACE('',(#2299),#950,.F.);
#22039=ADVANCED_FACE('',(#2300),#21808,.F.);
#22040=ADVANCED_FACE('',(#2301),#951,.F.);
#22041=ADVANCED_FACE('',(#2302),#21809,.F.);
#22042=ADVANCED_FACE('',(#2303),#952,.F.);
#22043=ADVANCED_FACE('',(#2304),#21810,.F.);
#22044=ADVANCED_FACE('',(#2305,#1291),#1475,.F.);
#22045=ADVANCED_FACE('',(#2306),#21811,.F.);
#22046=ADVANCED_FACE('',(#2307),#953,.F.);
#22047=ADVANCED_FACE('',(#2308),#21812,.F.);
#22048=ADVANCED_FACE('',(#2309,#1292),#1476,.F.);
#22049=ADVANCED_FACE('',(#2310),#21813,.F.);
#22050=ADVANCED_FACE('',(#2311),#954,.F.);
#22051=ADVANCED_FACE('',(#2312),#21814,.F.);
#22052=ADVANCED_FACE('',(#2313,#1293),#1477,.F.);
#22053=ADVANCED_FACE('',(#2314),#21815,.F.);
#22054=ADVANCED_FACE('',(#2315),#955,.F.);
#22055=ADVANCED_FACE('',(#2316),#21816,.F.);
#22056=ADVANCED_FACE('',(#2317,#1294),#1478,.F.);
#22057=ADVANCED_FACE('',(#2318),#21817,.F.);
#22058=ADVANCED_FACE('',(#2319),#956,.F.);
#22059=ADVANCED_FACE('',(#2320),#21818,.F.);
#22060=ADVANCED_FACE('',(#2321,#1295),#1479,.F.);
#22061=ADVANCED_FACE('',(#2322),#21819,.F.);
#22062=ADVANCED_FACE('',(#2323),#957,.F.);
#22063=ADVANCED_FACE('',(#2324),#21820,.F.);
#22064=ADVANCED_FACE('',(#2325,#1296),#1480,.F.);
#22065=ADVANCED_FACE('',(#2326),#21821,.F.);
#22066=ADVANCED_FACE('',(#2327),#958,.F.);
#22067=ADVANCED_FACE('',(#2328),#21822,.F.);
#22068=ADVANCED_FACE('',(#2329,#1297),#1481,.F.);
#22069=ADVANCED_FACE('',(#2330),#1482,.T.);
#22070=ADVANCED_FACE('',(#2331),#21823,.T.);
#22071=ADVANCED_FACE('',(#2332),#1483,.T.);
#22072=ADVANCED_FACE('',(#2333),#959,.T.);
#22073=ADVANCED_FACE('',(#2334),#960,.T.);
#22074=ADVANCED_FACE('',(#2335),#1484,.T.);
#23303=CLOSED_SHELL('',(#21975,#21976,#21977,#21978,#21979,#21980,#21981,
#21982,#21983,#21984,#21985,#21986,#21987,#21988,#21989,#21990,#21991,#21992,
#21993,#21994,#21995,#21996,#21997,#21998,#21999,#22000,#22001,#22002,#22003,
#22004,#22005,#22006,#22007,#22008,#22009,#22010,#22011,#22012,#22013,#22014,
#22015,#22016,#22017,#22018,#22019,#22020,#22021,#22022,#22023,#22024,#22025,
#22026,#22027,#22028,#22029,#22030,#22031,#22032,#22033,#22034,#22035,#22036,
#22037,#22038,#22039,#22040,#22041,#22042,#22043,#22044,#22045,#22046,#22047,
#22048,#22049,#22050,#22051,#22052,#22053,#22054,#22055,#22056,#22057,#22058,
#22059,#22060,#22061,#22062,#22063,#22064,#22065,#22066,#22067,#22068,#22069,
#22070,#22071,#22072,#22073,#22074));
#23497=AXIS2_PLACEMENT_3D('',#31816,#25656,#25657);
#23498=AXIS2_PLACEMENT_3D('',#31817,#25658,#25659);
#23499=AXIS2_PLACEMENT_3D('',#31822,#25661,#25662);
#23500=AXIS2_PLACEMENT_3D('',#31825,#25664,#25665);
#23501=AXIS2_PLACEMENT_3D('',#31826,#25666,#25667);
#23502=AXIS2_PLACEMENT_3D('',#31832,#25671,#25672);
#23503=AXIS2_PLACEMENT_3D('',#31836,#25674,#25675);
#23504=AXIS2_PLACEMENT_3D('',#31837,#25676,#25677);
#23505=AXIS2_PLACEMENT_3D('',#31838,#25678,#25679);
#23506=AXIS2_PLACEMENT_3D('',#31844,#25683,#25684);
#23507=AXIS2_PLACEMENT_3D('',#31848,#25686,#25687);
#23508=AXIS2_PLACEMENT_3D('',#31849,#25688,#25689);
#23509=AXIS2_PLACEMENT_3D('',#31850,#25690,#25691);
#23510=AXIS2_PLACEMENT_3D('',#31856,#25695,#25696);
#23511=AXIS2_PLACEMENT_3D('',#31860,#25698,#25699);
#23512=AXIS2_PLACEMENT_3D('',#31861,#25700,#25701);
#23513=AXIS2_PLACEMENT_3D('',#31862,#25702,#25703);
#23514=AXIS2_PLACEMENT_3D('',#31865,#25706,#25707);
#23515=AXIS2_PLACEMENT_3D('',#31871,#25711,#25712);
#23516=AXIS2_PLACEMENT_3D('',#31874,#25714,#25715);
#23517=AXIS2_PLACEMENT_3D('',#31875,#25716,#25717);
#23518=AXIS2_PLACEMENT_3D('',#31879,#25720,#25721);
#23519=AXIS2_PLACEMENT_3D('',#31882,#25723,#25724);
#23520=AXIS2_PLACEMENT_3D('',#31883,#25725,#25726);
#23521=AXIS2_PLACEMENT_3D('',#31885,#25727,#25728);
#23522=AXIS2_PLACEMENT_3D('',#31887,#25729,#25730);
#23523=AXIS2_PLACEMENT_3D('',#31889,#25731,#25732);
#23524=AXIS2_PLACEMENT_3D('',#31891,#25733,#25734);
#23525=AXIS2_PLACEMENT_3D('',#31893,#25735,#25736);
#23526=AXIS2_PLACEMENT_3D('',#31895,#25737,#25738);
#23527=AXIS2_PLACEMENT_3D('',#31897,#25739,#25740);
#23528=AXIS2_PLACEMENT_3D('',#31898,#25741,#25742);
#23529=AXIS2_PLACEMENT_3D('',#31903,#25745,#25746);
#23530=AXIS2_PLACEMENT_3D('',#31904,#25747,#25748);
#23531=AXIS2_PLACEMENT_3D('',#31908,#25751,#25752);
#23532=AXIS2_PLACEMENT_3D('',#31911,#25754,#25755);
#23533=AXIS2_PLACEMENT_3D('',#31912,#25756,#25757);
#23534=AXIS2_PLACEMENT_3D('',#31916,#25760,#25761);
#23535=AXIS2_PLACEMENT_3D('',#31920,#25763,#25764);
#23536=AXIS2_PLACEMENT_3D('',#31921,#25765,#25766);
#23537=AXIS2_PLACEMENT_3D('',#31922,#25767,#25768);
#23538=AXIS2_PLACEMENT_3D('',#31928,#25772,#25773);
#23539=AXIS2_PLACEMENT_3D('',#31932,#25775,#25776);
#23540=AXIS2_PLACEMENT_3D('',#31933,#25777,#25778);
#23541=AXIS2_PLACEMENT_3D('',#31934,#25779,#25780);
#23542=AXIS2_PLACEMENT_3D('',#31937,#25783,#25784);
#23543=AXIS2_PLACEMENT_3D('',#31943,#25788,#25789);
#23544=AXIS2_PLACEMENT_3D('',#31946,#25791,#25792);
#23545=AXIS2_PLACEMENT_3D('',#31947,#25793,#25794);
#23546=AXIS2_PLACEMENT_3D('',#31951,#25797,#25798);
#23547=AXIS2_PLACEMENT_3D('',#31954,#25800,#25801);
#23548=AXIS2_PLACEMENT_3D('',#31955,#25802,#25803);
#23549=AXIS2_PLACEMENT_3D('',#31958,#25806,#25807);
#23550=AXIS2_PLACEMENT_3D('',#31960,#25809,#25810);
#23551=AXIS2_PLACEMENT_3D('',#31961,#25811,#25812);
#23552=AXIS2_PLACEMENT_3D('',#31970,#25817,#25818);
#23553=AXIS2_PLACEMENT_3D('',#31974,#25820,#25821);
#23554=AXIS2_PLACEMENT_3D('',#31975,#25822,#25823);
#23555=AXIS2_PLACEMENT_3D('',#31976,#25824,#25825);
#23556=AXIS2_PLACEMENT_3D('',#31982,#25829,#25830);
#23557=AXIS2_PLACEMENT_3D('',#31986,#25832,#25833);
#23558=AXIS2_PLACEMENT_3D('',#31987,#25834,#25835);
#23559=AXIS2_PLACEMENT_3D('',#31988,#25836,#25837);
#23560=AXIS2_PLACEMENT_3D('',#31994,#25841,#25842);
#23561=AXIS2_PLACEMENT_3D('',#31998,#25844,#25845);
#23562=AXIS2_PLACEMENT_3D('',#31999,#25846,#25847);
#23563=AXIS2_PLACEMENT_3D('',#32000,#25848,#25849);
#23564=AXIS2_PLACEMENT_3D('',#32006,#25853,#25854);
#23565=AXIS2_PLACEMENT_3D('',#32007,#25855,#25856);
#23566=AXIS2_PLACEMENT_3D('',#32008,#25857,#25858);
#23567=AXIS2_PLACEMENT_3D('',#32009,#25859,#25860);
#23568=AXIS2_PLACEMENT_3D('',#32013,#25862,#25863);
#23569=AXIS2_PLACEMENT_3D('',#32015,#25865,#25866);
#23570=AXIS2_PLACEMENT_3D('',#32019,#25869,#25870);
#23571=AXIS2_PLACEMENT_3D('',#32022,#25872,#25873);
#23572=AXIS2_PLACEMENT_3D('',#32023,#25874,#25875);
#23573=AXIS2_PLACEMENT_3D('',#32027,#25878,#25879);
#23574=AXIS2_PLACEMENT_3D('',#32029,#25880,#25881);
#23575=AXIS2_PLACEMENT_3D('',#32031,#25882,#25883);
#23576=AXIS2_PLACEMENT_3D('',#32033,#25884,#25885);
#23577=AXIS2_PLACEMENT_3D('',#32035,#25886,#25887);
#23578=AXIS2_PLACEMENT_3D('',#32037,#25888,#25889);
#23579=AXIS2_PLACEMENT_3D('',#32039,#25890,#25891);
#23580=AXIS2_PLACEMENT_3D('',#32041,#25892,#25893);
#23581=AXIS2_PLACEMENT_3D('',#32042,#25894,#25895);
#23582=AXIS2_PLACEMENT_3D('',#32045,#25898,#25899);
#23583=AXIS2_PLACEMENT_3D('',#32047,#25901,#25902);
#23584=AXIS2_PLACEMENT_3D('',#32049,#25904,#25905);
#23585=AXIS2_PLACEMENT_3D('',#32051,#25907,#25908);
#23586=AXIS2_PLACEMENT_3D('',#32057,#25912,#25913);
#23587=AXIS2_PLACEMENT_3D('',#32061,#25915,#25916);
#23588=AXIS2_PLACEMENT_3D('',#32062,#25917,#25918);
#23589=AXIS2_PLACEMENT_3D('',#32063,#25919,#25920);
#23590=AXIS2_PLACEMENT_3D('',#32069,#25924,#25925);
#23591=AXIS2_PLACEMENT_3D('',#32070,#25926,#25927);
#23592=AXIS2_PLACEMENT_3D('',#32071,#25928,#25929);
#23593=AXIS2_PLACEMENT_3D('',#32072,#25930,#25931);
#23594=AXIS2_PLACEMENT_3D('',#32075,#25934,#25935);
#23595=AXIS2_PLACEMENT_3D('',#32077,#25937,#25938);
#23596=AXIS2_PLACEMENT_3D('',#32078,#25939,#25940);
#23597=AXIS2_PLACEMENT_3D('',#32082,#25942,#25943);
#23598=AXIS2_PLACEMENT_3D('',#32083,#25944,#25945);
#23599=AXIS2_PLACEMENT_3D('',#32084,#25946,#25947);
#23600=AXIS2_PLACEMENT_3D('',#32086,#25948,#25949);
#23601=AXIS2_PLACEMENT_3D('',#32088,#25951,#25952);
#23602=AXIS2_PLACEMENT_3D('',#32092,#25954,#25955);
#23603=AXIS2_PLACEMENT_3D('',#32093,#25956,#25957);
#23604=AXIS2_PLACEMENT_3D('',#32094,#25958,#25959);
#23605=AXIS2_PLACEMENT_3D('',#32096,#25960,#25961);
#23606=AXIS2_PLACEMENT_3D('',#32098,#25963,#25964);
#23607=AXIS2_PLACEMENT_3D('',#32102,#25966,#25967);
#23608=AXIS2_PLACEMENT_3D('',#32103,#25968,#25969);
#23609=AXIS2_PLACEMENT_3D('',#32104,#25970,#25971);
#23610=AXIS2_PLACEMENT_3D('',#32106,#25972,#25973);
#23611=AXIS2_PLACEMENT_3D('',#32108,#25975,#25976);
#23612=AXIS2_PLACEMENT_3D('',#32112,#25978,#25979);
#23613=AXIS2_PLACEMENT_3D('',#32113,#25980,#25981);
#23614=AXIS2_PLACEMENT_3D('',#32114,#25982,#25983);
#23615=AXIS2_PLACEMENT_3D('',#32116,#25984,#25985);
#23616=AXIS2_PLACEMENT_3D('',#32118,#25987,#25988);
#23617=AXIS2_PLACEMENT_3D('',#32122,#25990,#25991);
#23618=AXIS2_PLACEMENT_3D('',#32123,#25992,#25993);
#23619=AXIS2_PLACEMENT_3D('',#32124,#25994,#25995);
#23620=AXIS2_PLACEMENT_3D('',#32126,#25996,#25997);
#23621=AXIS2_PLACEMENT_3D('',#32128,#25999,#26000);
#23622=AXIS2_PLACEMENT_3D('',#32132,#26002,#26003);
#23623=AXIS2_PLACEMENT_3D('',#32133,#26004,#26005);
#23624=AXIS2_PLACEMENT_3D('',#32134,#26006,#26007);
#23625=AXIS2_PLACEMENT_3D('',#32136,#26008,#26009);
#23626=AXIS2_PLACEMENT_3D('',#32138,#26011,#26012);
#23627=AXIS2_PLACEMENT_3D('',#32142,#26014,#26015);
#23628=AXIS2_PLACEMENT_3D('',#32143,#26016,#26017);
#23629=AXIS2_PLACEMENT_3D('',#32144,#26018,#26019);
#23630=AXIS2_PLACEMENT_3D('',#32146,#26020,#26021);
#23631=AXIS2_PLACEMENT_3D('',#32148,#26023,#26024);
#23632=AXIS2_PLACEMENT_3D('',#32151,#26026,#26027);
#23633=AXIS2_PLACEMENT_3D('',#32152,#26028,#26029);
#23634=AXIS2_PLACEMENT_3D('',#32155,#26031,#26032);
#23635=AXIS2_PLACEMENT_3D('',#32156,#26033,#26034);
#23636=AXIS2_PLACEMENT_3D('',#32159,#26036,#26037);
#23637=AXIS2_PLACEMENT_3D('',#32160,#26038,#26039);
#23638=AXIS2_PLACEMENT_3D('',#32161,#26040,#26041);
#23639=AXIS2_PLACEMENT_3D('',#32164,#26043,#26044);
#23640=AXIS2_PLACEMENT_3D('',#32165,#26045,#26046);
#23641=AXIS2_PLACEMENT_3D('',#32168,#26048,#26049);
#23642=AXIS2_PLACEMENT_3D('',#32169,#26050,#26051);
#23643=AXIS2_PLACEMENT_3D('',#32172,#26053,#26054);
#23644=AXIS2_PLACEMENT_3D('',#32173,#26055,#26056);
#23645=AXIS2_PLACEMENT_3D('',#32174,#26057,#26058);
#23646=AXIS2_PLACEMENT_3D('',#32177,#26060,#26061);
#23647=AXIS2_PLACEMENT_3D('',#32178,#26062,#26063);
#23648=AXIS2_PLACEMENT_3D('',#32181,#26065,#26066);
#23649=AXIS2_PLACEMENT_3D('',#32182,#26067,#26068);
#23650=AXIS2_PLACEMENT_3D('',#32185,#26070,#26071);
#23651=AXIS2_PLACEMENT_3D('',#32186,#26072,#26073);
#23652=AXIS2_PLACEMENT_3D('',#32187,#26074,#26075);
#23653=AXIS2_PLACEMENT_3D('',#32190,#26077,#26078);
#23654=AXIS2_PLACEMENT_3D('',#32191,#26079,#26080);
#23655=AXIS2_PLACEMENT_3D('',#32194,#26082,#26083);
#23656=AXIS2_PLACEMENT_3D('',#32195,#26084,#26085);
#23657=AXIS2_PLACEMENT_3D('',#32198,#26087,#26088);
#23658=AXIS2_PLACEMENT_3D('',#32199,#26089,#26090);
#23659=AXIS2_PLACEMENT_3D('',#32200,#26091,#26092);
#23660=AXIS2_PLACEMENT_3D('',#32203,#26094,#26095);
#23661=AXIS2_PLACEMENT_3D('',#32204,#26096,#26097);
#23662=AXIS2_PLACEMENT_3D('',#32207,#26099,#26100);
#23663=AXIS2_PLACEMENT_3D('',#32208,#26101,#26102);
#23664=AXIS2_PLACEMENT_3D('',#32211,#26104,#26105);
#23665=AXIS2_PLACEMENT_3D('',#32212,#26106,#26107);
#23666=AXIS2_PLACEMENT_3D('',#32213,#26108,#26109);
#23667=AXIS2_PLACEMENT_3D('',#32216,#26111,#26112);
#23668=AXIS2_PLACEMENT_3D('',#32217,#26113,#26114);
#23669=AXIS2_PLACEMENT_3D('',#32220,#26116,#26117);
#23670=AXIS2_PLACEMENT_3D('',#32221,#26118,#26119);
#23671=AXIS2_PLACEMENT_3D('',#32224,#26121,#26122);
#23672=AXIS2_PLACEMENT_3D('',#32225,#26123,#26124);
#23673=AXIS2_PLACEMENT_3D('',#32226,#26125,#26126);
#23674=AXIS2_PLACEMENT_3D('',#32229,#26128,#26129);
#23675=AXIS2_PLACEMENT_3D('',#32230,#26130,#26131);
#23676=AXIS2_PLACEMENT_3D('',#32233,#26133,#26134);
#23677=AXIS2_PLACEMENT_3D('',#32234,#26135,#26136);
#23678=AXIS2_PLACEMENT_3D('',#32237,#26138,#26139);
#23679=AXIS2_PLACEMENT_3D('',#32238,#26140,#26141);
#23680=AXIS2_PLACEMENT_3D('',#32239,#26142,#26143);
#23681=AXIS2_PLACEMENT_3D('',#32240,#26144,#26145);
#23682=AXIS2_PLACEMENT_3D('',#32241,#26146,#26147);
#23683=AXIS2_PLACEMENT_3D('',#32243,#26149,#26150);
#23684=AXIS2_PLACEMENT_3D('',#32245,#26152,#26153);
#23685=AXIS2_PLACEMENT_3D('',#32247,#26155,#26156);
#25656=DIRECTION('axis',(0.,0.,1.));
#25657=DIRECTION('refdir',(1.,0.,0.));
#25658=DIRECTION('center_axis',(0.,0.,-1.));
#25659=DIRECTION('ref_axis',(-0.707106781186548,-0.707106781186548,0.));
#25660=DIRECTION('',(-0.923879532511286,0.,-0.382683432365092));
#25661=DIRECTION('center_axis',(0.,0.,1.));
#25662=DIRECTION('ref_axis',(-0.707106781186547,-0.707106781186547,0.));
#25663=DIRECTION('',(0.,0.923879532511286,0.382683432365092));
#25664=DIRECTION('center_axis',(0.,0.,-1.));
#25665=DIRECTION('ref_axis',(-0.707106781186547,-0.707106781186547,0.));
#25666=DIRECTION('center_axis',(-0.382683432365103,0.,0.923879532511281));
#25667=DIRECTION('ref_axis',(0.923879532511281,0.,0.382683432365103));
#25668=DIRECTION('',(-0.923879532511283,0.,-0.3826834323651));
#25669=DIRECTION('',(0.,-1.,0.));
#25670=DIRECTION('',(0.,1.,0.));
#25671=DIRECTION('center_axis',(0.,0.,-1.));
#25672=DIRECTION('ref_axis',(-0.707106781186548,0.707106781186548,0.));
#25673=DIRECTION('',(0.,0.923879532511286,-0.382683432365092));
#25674=DIRECTION('center_axis',(0.,0.,1.));
#25675=DIRECTION('ref_axis',(-0.707106781186547,0.707106781186547,0.));
#25676=DIRECTION('center_axis',(0.,0.,-1.));
#25677=DIRECTION('ref_axis',(-0.707106781186547,0.707106781186547,0.));
#25678=DIRECTION('center_axis',(0.,0.382683432365094,0.923879532511285));
#25679=DIRECTION('ref_axis',(1.,0.,0.));
#25680=DIRECTION('',(0.,0.923879532511285,-0.382683432365094));
#25681=DIRECTION('',(-1.,0.,0.));
#25682=DIRECTION('',(1.,0.,0.));
#25683=DIRECTION('center_axis',(0.,0.,-1.));
#25684=DIRECTION('ref_axis',(0.707106781186548,0.707106781186548,0.));
#25685=DIRECTION('',(0.923879532511286,0.,-0.382683432365092));
#25686=DIRECTION('center_axis',(0.,0.,1.));
#25687=DIRECTION('ref_axis',(0.707106781186547,0.707106781186547,0.));
#25688=DIRECTION('center_axis',(0.,0.,-1.));
#25689=DIRECTION('ref_axis',(0.707106781186547,0.707106781186547,0.));
#25690=DIRECTION('center_axis',(0.382683432365103,0.,0.923879532511281));
#25691=DIRECTION('ref_axis',(0.923879532511281,0.,-0.382683432365103));
#25692=DIRECTION('',(0.923879532511283,0.,-0.3826834323651));
#25693=DIRECTION('',(0.,1.,0.));
#25694=DIRECTION('',(0.,-1.,0.));
#25695=DIRECTION('center_axis',(0.,0.,-1.));
#25696=DIRECTION('ref_axis',(0.707106781186548,-0.707106781186548,0.));
#25697=DIRECTION('',(0.,-0.923879532511286,-0.382683432365092));
#25698=DIRECTION('center_axis',(0.,0.,1.));
#25699=DIRECTION('ref_axis',(0.707106781186547,-0.707106781186547,0.));
#25700=DIRECTION('center_axis',(0.,0.,-1.));
#25701=DIRECTION('ref_axis',(0.707106781186547,-0.707106781186547,0.));
#25702=DIRECTION('center_axis',(0.,-0.382683432365094,0.923879532511285));
#25703=DIRECTION('ref_axis',(1.,0.,0.));
#25704=DIRECTION('',(1.,0.,0.));
#25705=DIRECTION('',(-1.,0.,0.));
#25706=DIRECTION('center_axis',(0.707106781186549,0.,0.707106781186546));
#25707=DIRECTION('ref_axis',(0.707106781186546,0.,-0.707106781186549));
#25708=DIRECTION('',(0.707106781186546,0.,-0.707106781186549));
#25709=DIRECTION('',(0.,-1.,0.));
#25710=DIRECTION('',(0.707106781186546,0.,-0.707106781186549));
#25711=DIRECTION('center_axis',(0.,0.,-1.));
#25712=DIRECTION('ref_axis',(0.707106781186548,-0.707106781186548,0.));
#25713=DIRECTION('',(0.,-0.707106781186546,-0.707106781186549));
#25714=DIRECTION('center_axis',(0.,0.,-1.));
#25715=DIRECTION('ref_axis',(0.707106781186547,-0.707106781186547,0.));
#25716=DIRECTION('center_axis',(0.,-0.707106781186549,0.707106781186546));
#25717=DIRECTION('ref_axis',(1.,0.,0.));
#25718=DIRECTION('',(0.,0.707106781186546,0.707106781186549));
#25719=DIRECTION('',(-1.,0.,0.));
#25720=DIRECTION('center_axis',(0.,0.,-1.));
#25721=DIRECTION('ref_axis',(-0.707106781186548,-0.707106781186548,0.));
#25722=DIRECTION('',(-0.707106781186546,0.,-0.707106781186549));
#25723=DIRECTION('center_axis',(0.,0.,-1.));
#25724=DIRECTION('ref_axis',(-0.707106781186547,-0.707106781186547,0.));
#25725=DIRECTION('center_axis',(0.,0.,1.));
#25726=DIRECTION('ref_axis',(1.,0.,0.));
#25727=DIRECTION('center_axis',(0.,0.,1.));
#25728=DIRECTION('ref_axis',(-1.,0.,0.));
#25729=DIRECTION('center_axis',(0.,0.,1.));
#25730=DIRECTION('ref_axis',(-1.,0.,0.));
#25731=DIRECTION('center_axis',(0.,0.,-1.));
#25732=DIRECTION('ref_axis',(-1.,0.,0.));
#25733=DIRECTION('center_axis',(0.,0.,-1.));
#25734=DIRECTION('ref_axis',(-1.,0.,0.));
#25735=DIRECTION('center_axis',(0.,0.,-1.));
#25736=DIRECTION('ref_axis',(-1.,0.,0.));
#25737=DIRECTION('center_axis',(0.,0.,1.));
#25738=DIRECTION('ref_axis',(-1.,0.,0.));
#25739=DIRECTION('center_axis',(0.,0.,1.));
#25740=DIRECTION('ref_axis',(-1.,0.,0.));
#25741=DIRECTION('center_axis',(0.,0.,-1.));
#25742=DIRECTION('ref_axis',(-0.707106781186547,-0.707106781186547,0.));
#25743=DIRECTION('',(0.,0.382683432365082,0.92387953251129));
#25744=DIRECTION('',(-0.382683432365082,0.,-0.92387953251129));
#25745=DIRECTION('center_axis',(0.,0.,1.));
#25746=DIRECTION('ref_axis',(-0.707106781186547,-0.707106781186547,0.));
#25747=DIRECTION('center_axis',(0.,-0.923879532511285,0.382683432365094));
#25748=DIRECTION('ref_axis',(0.,-0.382683432365094,-0.923879532511285));
#25749=DIRECTION('',(0.,0.382683432365095,0.923879532511285));
#25750=DIRECTION('',(1.,0.,0.));
#25751=DIRECTION('center_axis',(0.,0.,-1.));
#25752=DIRECTION('ref_axis',(0.707106781186547,-0.707106781186547,0.));
#25753=DIRECTION('',(-0.382683432365082,0.,0.92387953251129));
#25754=DIRECTION('center_axis',(0.,0.,1.));
#25755=DIRECTION('ref_axis',(0.707106781186547,-0.707106781186547,0.));
#25756=DIRECTION('center_axis',(0.923879532511285,0.,0.382683432365094));
#25757=DIRECTION('ref_axis',(0.382683432365094,0.,-0.923879532511285));
#25758=DIRECTION('',(-0.382683432365095,0.,0.923879532511285));
#25759=DIRECTION('',(0.,1.,0.));
#25760=DIRECTION('center_axis',(0.,0.,-1.));
#25761=DIRECTION('ref_axis',(0.707106781186547,0.707106781186547,0.));
#25762=DIRECTION('',(0.,-0.382683432365082,0.92387953251129));
#25763=DIRECTION('center_axis',(0.,0.,-1.));
#25764=DIRECTION('ref_axis',(0.707106781186547,0.707106781186547,0.));
#25765=DIRECTION('center_axis',(0.,0.,1.));
#25766=DIRECTION('ref_axis',(0.707106781186547,0.707106781186547,0.));
#25767=DIRECTION('center_axis',(0.,0.923879532511285,0.382683432365094));
#25768=DIRECTION('ref_axis',(0.,-0.382683432365094,0.923879532511285));
#25769=DIRECTION('',(0.,-0.382683432365095,0.923879532511285));
#25770=DIRECTION('',(1.,0.,0.));
#25771=DIRECTION('',(-1.,0.,0.));
#25772=DIRECTION('center_axis',(0.,0.,-1.));
#25773=DIRECTION('ref_axis',(-0.707106781186547,0.707106781186547,0.));
#25774=DIRECTION('',(0.382683432365082,0.,0.92387953251129));
#25775=DIRECTION('center_axis',(0.,0.,-1.));
#25776=DIRECTION('ref_axis',(-0.707106781186547,0.707106781186547,0.));
#25777=DIRECTION('center_axis',(0.,0.,1.));
#25778=DIRECTION('ref_axis',(-0.707106781186547,0.707106781186547,0.));
#25779=DIRECTION('center_axis',(-0.923879532511285,0.,0.382683432365094));
#25780=DIRECTION('ref_axis',(0.382683432365094,0.,0.923879532511285));
#25781=DIRECTION('',(0.,1.,0.));
#25782=DIRECTION('',(0.,-1.,0.));
#25783=DIRECTION('center_axis',(1.,0.,0.));
#25784=DIRECTION('ref_axis',(0.,1.,0.));
#25785=DIRECTION('',(0.,0.,1.));
#25786=DIRECTION('',(0.,-1.,0.));
#25787=DIRECTION('',(0.,0.,-1.));
#25788=DIRECTION('center_axis',(0.,0.,1.));
#25789=DIRECTION('ref_axis',(0.707106781186547,-0.707106781186547,0.));
#25790=DIRECTION('',(0.,0.,-1.));
#25791=DIRECTION('center_axis',(0.,0.,-1.));
#25792=DIRECTION('ref_axis',(0.707106781186547,-0.707106781186547,0.));
#25793=DIRECTION('center_axis',(0.,-1.,0.));
#25794=DIRECTION('ref_axis',(1.,0.,0.));
#25795=DIRECTION('',(0.,0.,1.));
#25796=DIRECTION('',(-1.,0.,0.));
#25797=DIRECTION('center_axis',(0.,0.,1.));
#25798=DIRECTION('ref_axis',(-0.707106781186547,-0.707106781186547,0.));
#25799=DIRECTION('',(0.,0.,-1.));
#25800=DIRECTION('center_axis',(0.,0.,-1.));
#25801=DIRECTION('ref_axis',(-0.707106781186547,-0.707106781186547,0.));
#25802=DIRECTION('center_axis',(0.,0.707106781186549,0.707106781186546));
#25803=DIRECTION('ref_axis',(1.,0.,0.));
#25804=DIRECTION('',(0.,0.707106781186546,-0.707106781186549));
#25805=DIRECTION('',(0.,0.707106781186546,-0.707106781186549));
#25806=DIRECTION('center_axis',(0.,0.,-1.));
#25807=DIRECTION('ref_axis',(-0.707106781186548,0.707106781186548,0.));
#25808=DIRECTION('',(-0.707106781186546,0.,-0.707106781186549));
#25809=DIRECTION('center_axis',(-0.707106781186549,0.,0.707106781186546));
#25810=DIRECTION('ref_axis',(0.707106781186546,0.,0.707106781186549));
#25811=DIRECTION('center_axis',(0.38268343236509,0.,-0.923879532511287));
#25812=DIRECTION('ref_axis',(-0.923879532511287,0.,-0.38268343236509));
#25813=DIRECTION('',(0.923879532511288,0.,0.382683432365087));
#25814=DIRECTION('',(0.,-1.,0.));
#25815=DIRECTION('',(-0.923879532511288,0.,-0.382683432365087));
#25816=DIRECTION('',(0.,1.,0.));
#25817=DIRECTION('center_axis',(0.,0.,1.));
#25818=DIRECTION('ref_axis',(0.707106781186548,0.707106781186548,0.));
#25819=DIRECTION('',(0.,0.923879532511292,0.382683432365076));
#25820=DIRECTION('center_axis',(0.,0.,-1.));
#25821=DIRECTION('ref_axis',(0.707106781186548,0.707106781186548,0.));
#25822=DIRECTION('center_axis',(0.,0.,1.));
#25823=DIRECTION('ref_axis',(0.707106781186548,0.707106781186548,0.));
#25824=DIRECTION('center_axis',(0.,0.382683432365092,-0.923879532511286));
#25825=DIRECTION('ref_axis',(-1.,0.,0.));
#25826=DIRECTION('',(0.,0.923879532511288,0.382683432365088));
#25827=DIRECTION('',(1.,0.,0.));
#25828=DIRECTION('',(-1.,0.,0.));
#25829=DIRECTION('center_axis',(0.,0.,1.));
#25830=DIRECTION('ref_axis',(-0.707106781186548,0.707106781186548,0.));
#25831=DIRECTION('',(-0.923879532511292,0.,0.382683432365076));
#25832=DIRECTION('center_axis',(0.,0.,-1.));
#25833=DIRECTION('ref_axis',(-0.707106781186548,0.707106781186548,0.));
#25834=DIRECTION('center_axis',(0.,0.,1.));
#25835=DIRECTION('ref_axis',(-0.707106781186548,0.707106781186548,0.));
#25836=DIRECTION('center_axis',(-0.38268343236509,0.,-0.923879532511287));
#25837=DIRECTION('ref_axis',(-0.923879532511287,0.,0.38268343236509));
#25838=DIRECTION('',(-0.923879532511288,0.,0.382683432365087));
#25839=DIRECTION('',(0.,1.,0.));
#25840=DIRECTION('',(0.,-1.,0.));
#25841=DIRECTION('center_axis',(0.,0.,1.));
#25842=DIRECTION('ref_axis',(-0.707106781186548,-0.707106781186548,0.));
#25843=DIRECTION('',(0.,-0.923879532511292,0.382683432365076));
#25844=DIRECTION('center_axis',(0.,0.,-1.));
#25845=DIRECTION('ref_axis',(-0.707106781186548,-0.707106781186548,0.));
#25846=DIRECTION('center_axis',(0.,0.,1.));
#25847=DIRECTION('ref_axis',(-0.707106781186548,-0.707106781186548,0.));
#25848=DIRECTION('center_axis',(0.,-0.382683432365092,-0.923879532511286));
#25849=DIRECTION('ref_axis',(-1.,0.,0.));
#25850=DIRECTION('',(0.,-0.923879532511288,0.382683432365088));
#25851=DIRECTION('',(-1.,0.,0.));
#25852=DIRECTION('',(1.,0.,0.));
#25853=DIRECTION('center_axis',(0.,0.,1.));
#25854=DIRECTION('ref_axis',(0.707106781186548,-0.707106781186548,0.));
#25855=DIRECTION('center_axis',(0.,0.,-1.));
#25856=DIRECTION('ref_axis',(0.707106781186548,-0.707106781186548,0.));
#25857=DIRECTION('center_axis',(0.,0.,1.));
#25858=DIRECTION('ref_axis',(0.707106781186548,-0.707106781186548,0.));
#25859=DIRECTION('center_axis',(0.,0.,1.));
#25860=DIRECTION('ref_axis',(-0.707106781186548,-0.707106781186548,0.));
#25861=DIRECTION('',(0.,-0.70710678118654,0.707106781186555));
#25862=DIRECTION('center_axis',(0.,0.,1.));
#25863=DIRECTION('ref_axis',(-0.707106781186547,-0.707106781186547,0.));
#25864=DIRECTION('',(-0.707106781186546,0.,0.707106781186549));
#25865=DIRECTION('center_axis',(0.,-0.707106781186549,-0.707106781186546));
#25866=DIRECTION('ref_axis',(-1.,0.,0.));
#25867=DIRECTION('',(0.,-0.707106781186546,0.707106781186549));
#25868=DIRECTION('',(1.,0.,0.));
#25869=DIRECTION('center_axis',(0.,0.,1.));
#25870=DIRECTION('ref_axis',(0.707106781186548,-0.707106781186548,0.));
#25871=DIRECTION('',(-0.707106781186546,0.,-0.707106781186549));
#25872=DIRECTION('center_axis',(0.,0.,1.));
#25873=DIRECTION('ref_axis',(0.707106781186547,-0.707106781186547,0.));
#25874=DIRECTION('center_axis',(0.707106781186549,0.,-0.707106781186546));
#25875=DIRECTION('ref_axis',(-0.707106781186546,0.,-0.707106781186549));
#25876=DIRECTION('',(0.707106781186546,0.,0.707106781186549));
#25877=DIRECTION('',(0.,1.,0.));
#25878=DIRECTION('center_axis',(0.,0.,1.));
#25879=DIRECTION('ref_axis',(1.,0.,0.));
#25880=DIRECTION('center_axis',(0.,0.,-1.));
#25881=DIRECTION('ref_axis',(1.,0.,0.));
#25882=DIRECTION('center_axis',(0.,0.,-1.));
#25883=DIRECTION('ref_axis',(1.,0.,0.));
#25884=DIRECTION('center_axis',(0.,0.,1.));
#25885=DIRECTION('ref_axis',(1.,0.,0.));
#25886=DIRECTION('center_axis',(0.,0.,1.));
#25887=DIRECTION('ref_axis',(1.,0.,0.));
#25888=DIRECTION('center_axis',(0.,0.,1.));
#25889=DIRECTION('ref_axis',(1.,0.,0.));
#25890=DIRECTION('center_axis',(0.,0.,1.));
#25891=DIRECTION('ref_axis',(1.,0.,0.));
#25892=DIRECTION('center_axis',(0.,0.,-1.));
#25893=DIRECTION('ref_axis',(1.,0.,0.));
#25894=DIRECTION('center_axis',(0.923879532511292,0.,-0.382683432365078));
#25895=DIRECTION('ref_axis',(-0.382683432365078,0.,-0.923879532511292));
#25896=DIRECTION('',(-0.382683432365076,0.,-0.923879532511293));
#25897=DIRECTION('',(0.382683432365076,0.,0.923879532511293));
#25898=DIRECTION('center_axis',(0.,0.,1.));
#25899=DIRECTION('ref_axis',(0.707106781186547,-0.707106781186547,0.));
#25900=DIRECTION('',(0.,0.382683432365084,-0.923879532511289));
#25901=DIRECTION('center_axis',(0.,-0.923879532511292,-0.382683432365078));
#25902=DIRECTION('ref_axis',(0.,0.382683432365078,-0.923879532511292));
#25903=DIRECTION('',(0.,0.382683432365061,-0.923879532511299));
#25904=DIRECTION('center_axis',(0.,0.,1.));
#25905=DIRECTION('ref_axis',(-0.707106781186547,-0.707106781186547,0.));
#25906=DIRECTION('',(0.382683432365084,0.,-0.923879532511289));
#25907=DIRECTION('center_axis',(-0.923879532511292,0.,-0.382683432365078));
#25908=DIRECTION('ref_axis',(-0.382683432365078,0.,0.923879532511292));
#25909=DIRECTION('',(0.382683432365061,0.,-0.923879532511299));
#25910=DIRECTION('',(0.,-1.,0.));
#25911=DIRECTION('',(0.,1.,0.));
#25912=DIRECTION('center_axis',(0.,0.,1.));
#25913=DIRECTION('ref_axis',(-0.707106781186547,0.707106781186547,0.));
#25914=DIRECTION('',(0.,-0.382683432365084,-0.923879532511289));
#25915=DIRECTION('center_axis',(0.,0.,1.));
#25916=DIRECTION('ref_axis',(-0.707106781186547,0.707106781186547,0.));
#25917=DIRECTION('center_axis',(0.,0.,-1.));
#25918=DIRECTION('ref_axis',(-0.707106781186547,0.707106781186547,0.));
#25919=DIRECTION('center_axis',(0.,0.923879532511292,-0.382683432365078));
#25920=DIRECTION('ref_axis',(0.,0.382683432365078,0.923879532511292));
#25921=DIRECTION('',(0.,-0.382683432365061,-0.923879532511299));
#25922=DIRECTION('',(-1.,0.,0.));
#25923=DIRECTION('',(1.,0.,0.));
#25924=DIRECTION('center_axis',(0.,0.,1.));
#25925=DIRECTION('ref_axis',(0.707106781186547,0.707106781186547,0.));
#25926=DIRECTION('center_axis',(0.,0.,1.));
#25927=DIRECTION('ref_axis',(0.707106781186547,0.707106781186547,0.));
#25928=DIRECTION('center_axis',(0.,0.,-1.));
#25929=DIRECTION('ref_axis',(0.707106781186547,0.707106781186547,0.));
#25930=DIRECTION('center_axis',(0.,0.,1.));
#25931=DIRECTION('ref_axis',(-0.707106781186548,0.707106781186548,0.));
#25932=DIRECTION('',(-0.70710678118654,0.,0.707106781186555));
#25933=DIRECTION('',(0.,0.707106781186546,0.707106781186549));
#25934=DIRECTION('center_axis',(0.,0.707106781186549,-0.707106781186546));
#25935=DIRECTION('ref_axis',(-1.,0.,0.));
#25936=DIRECTION('',(0.,0.70710678118654,0.707106781186555));
#25937=DIRECTION('center_axis',(0.,0.,1.));
#25938=DIRECTION('ref_axis',(0.707106781186548,0.707106781186548,0.));
#25939=DIRECTION('center_axis',(0.,0.,1.));
#25940=DIRECTION('ref_axis',(-1.,0.,0.));
#25941=DIRECTION('',(-0.70710678118655,-8.65956056235496E-17,-0.707106781186545));
#25942=DIRECTION('center_axis',(0.,0.,-1.));
#25943=DIRECTION('ref_axis',(-1.,0.,0.));
#25944=DIRECTION('center_axis',(0.,0.,-1.));
#25945=DIRECTION('ref_axis',(-1.,0.,0.));
#25946=DIRECTION('center_axis',(0.,0.,1.));
#25947=DIRECTION('ref_axis',(1.,0.,0.));
#25948=DIRECTION('center_axis',(0.,0.,1.));
#25949=DIRECTION('ref_axis',(1.,0.,0.));
#25950=DIRECTION('',(0.,0.,1.));
#25951=DIRECTION('center_axis',(0.,0.,1.));
#25952=DIRECTION('ref_axis',(-1.,0.,0.));
#25953=DIRECTION('',(-0.70710678118655,-8.65956056235496E-17,-0.707106781186545));
#25954=DIRECTION('center_axis',(0.,0.,-1.));
#25955=DIRECTION('ref_axis',(-1.,0.,0.));
#25956=DIRECTION('center_axis',(0.,0.,-1.));
#25957=DIRECTION('ref_axis',(-1.,0.,0.));
#25958=DIRECTION('center_axis',(0.,0.,1.));
#25959=DIRECTION('ref_axis',(1.,0.,0.));
#25960=DIRECTION('center_axis',(0.,0.,1.));
#25961=DIRECTION('ref_axis',(1.,0.,0.));
#25962=DIRECTION('',(0.,0.,1.));
#25963=DIRECTION('center_axis',(0.,0.,1.));
#25964=DIRECTION('ref_axis',(-1.,0.,0.));
#25965=DIRECTION('',(-0.70710678118655,-8.65956056235496E-17,-0.707106781186545));
#25966=DIRECTION('center_axis',(0.,0.,-1.));
#25967=DIRECTION('ref_axis',(-1.,0.,0.));
#25968=DIRECTION('center_axis',(0.,0.,-1.));
#25969=DIRECTION('ref_axis',(-1.,0.,0.));
#25970=DIRECTION('center_axis',(0.,0.,1.));
#25971=DIRECTION('ref_axis',(1.,0.,0.));
#25972=DIRECTION('center_axis',(0.,0.,1.));
#25973=DIRECTION('ref_axis',(1.,0.,0.));
#25974=DIRECTION('',(0.,0.,1.));
#25975=DIRECTION('center_axis',(0.,0.,1.));
#25976=DIRECTION('ref_axis',(-1.,0.,0.));
#25977=DIRECTION('',(-0.70710678118655,-8.65956056235496E-17,-0.707106781186545));
#25978=DIRECTION('center_axis',(0.,0.,-1.));
#25979=DIRECTION('ref_axis',(-1.,0.,0.));
#25980=DIRECTION('center_axis',(0.,0.,-1.));
#25981=DIRECTION('ref_axis',(-1.,0.,0.));
#25982=DIRECTION('center_axis',(0.,0.,1.));
#25983=DIRECTION('ref_axis',(1.,0.,0.));
#25984=DIRECTION('center_axis',(0.,0.,1.));
#25985=DIRECTION('ref_axis',(1.,0.,0.));
#25986=DIRECTION('',(0.,0.,1.));
#25987=DIRECTION('center_axis',(0.,0.,-1.));
#25988=DIRECTION('ref_axis',(1.,0.,0.));
#25989=DIRECTION('',(0.707106781186545,-8.6595605623549E-17,0.70710678118655));
#25990=DIRECTION('center_axis',(0.,0.,1.));
#25991=DIRECTION('ref_axis',(1.,0.,0.));
#25992=DIRECTION('center_axis',(0.,0.,1.));
#25993=DIRECTION('ref_axis',(1.,0.,0.));
#25994=DIRECTION('center_axis',(0.,0.,-1.));
#25995=DIRECTION('ref_axis',(-1.,0.,0.));
#25996=DIRECTION('center_axis',(0.,0.,-1.));
#25997=DIRECTION('ref_axis',(1.,0.,0.));
#25998=DIRECTION('',(0.,0.,-1.));
#25999=DIRECTION('center_axis',(0.,0.,-1.));
#26000=DIRECTION('ref_axis',(1.,0.,0.));
#26001=DIRECTION('',(0.707106781186548,-8.65956056235494E-17,0.707106781186547));
#26002=DIRECTION('center_axis',(0.,0.,1.));
#26003=DIRECTION('ref_axis',(1.,0.,0.));
#26004=DIRECTION('center_axis',(0.,0.,1.));
#26005=DIRECTION('ref_axis',(1.,0.,0.));
#26006=DIRECTION('center_axis',(0.,0.,-1.));
#26007=DIRECTION('ref_axis',(-1.,0.,0.));
#26008=DIRECTION('center_axis',(0.,0.,-1.));
#26009=DIRECTION('ref_axis',(1.,0.,0.));
#26010=DIRECTION('',(0.,0.,-1.));
#26011=DIRECTION('center_axis',(0.,0.,-1.));
#26012=DIRECTION('ref_axis',(1.,0.,0.));
#26013=DIRECTION('',(0.70710678118655,-8.65956056235497E-17,0.707106781186545));
#26014=DIRECTION('center_axis',(0.,0.,1.));
#26015=DIRECTION('ref_axis',(1.,0.,0.));
#26016=DIRECTION('center_axis',(0.,0.,1.));
#26017=DIRECTION('ref_axis',(1.,0.,0.));
#26018=DIRECTION('center_axis',(0.,0.,-1.));
#26019=DIRECTION('ref_axis',(-1.,0.,0.));
#26020=DIRECTION('center_axis',(0.,0.,-1.));
#26021=DIRECTION('ref_axis',(1.,0.,0.));
#26022=DIRECTION('',(0.,0.,-1.));
#26023=DIRECTION('center_axis',(0.,0.,1.));
#26024=DIRECTION('ref_axis',(-1.,0.,0.));
#26025=DIRECTION('',(-0.316227766016832,3.87267321454032E-17,-0.948683298050516));
#26026=DIRECTION('center_axis',(0.,0.,-1.));
#26027=DIRECTION('ref_axis',(1.,0.,0.));
#26028=DIRECTION('center_axis',(0.,0.,-1.));
#26029=DIRECTION('ref_axis',(-1.,0.,0.));
#26030=DIRECTION('',(0.,0.,-1.));
#26031=DIRECTION('center_axis',(0.,0.,-1.));
#26032=DIRECTION('ref_axis',(1.,0.,0.));
#26033=DIRECTION('center_axis',(0.,0.,-1.));
#26034=DIRECTION('ref_axis',(-1.,0.,0.));
#26035=DIRECTION('',(0.707106781186541,-8.65956056235486E-17,-0.707106781186554));
#26036=DIRECTION('center_axis',(0.,0.,-1.));
#26037=DIRECTION('ref_axis',(1.,0.,0.));
#26038=DIRECTION('center_axis',(0.,0.,1.));
#26039=DIRECTION('ref_axis',(1.,0.,0.));
#26040=DIRECTION('center_axis',(0.,0.,1.));
#26041=DIRECTION('ref_axis',(-1.,0.,0.));
#26042=DIRECTION('',(-0.316227766016838,3.87267321454038E-17,-0.948683298050514));
#26043=DIRECTION('center_axis',(0.,0.,-1.));
#26044=DIRECTION('ref_axis',(1.,0.,0.));
#26045=DIRECTION('center_axis',(0.,0.,-1.));
#26046=DIRECTION('ref_axis',(-1.,0.,0.));
#26047=DIRECTION('',(0.,0.,-1.));
#26048=DIRECTION('center_axis',(0.,0.,-1.));
#26049=DIRECTION('ref_axis',(1.,0.,0.));
#26050=DIRECTION('center_axis',(0.,0.,-1.));
#26051=DIRECTION('ref_axis',(-1.,0.,0.));
#26052=DIRECTION('',(0.707106781186548,-8.65956056235494E-17,-0.707106781186547));
#26053=DIRECTION('center_axis',(0.,0.,-1.));
#26054=DIRECTION('ref_axis',(1.,0.,0.));
#26055=DIRECTION('center_axis',(0.,0.,1.));
#26056=DIRECTION('ref_axis',(1.,0.,0.));
#26057=DIRECTION('center_axis',(0.,0.,1.));
#26058=DIRECTION('ref_axis',(-1.,0.,0.));
#26059=DIRECTION('',(-0.316227766016832,3.87267321454032E-17,-0.948683298050516));
#26060=DIRECTION('center_axis',(0.,0.,-1.));
#26061=DIRECTION('ref_axis',(1.,0.,0.));
#26062=DIRECTION('center_axis',(0.,0.,-1.));
#26063=DIRECTION('ref_axis',(-1.,0.,0.));
#26064=DIRECTION('',(0.,0.,-1.));
#26065=DIRECTION('center_axis',(0.,0.,-1.));
#26066=DIRECTION('ref_axis',(1.,0.,0.));
#26067=DIRECTION('center_axis',(0.,0.,-1.));
#26068=DIRECTION('ref_axis',(-1.,0.,0.));
#26069=DIRECTION('',(0.707106781186541,-8.65956056235486E-17,-0.707106781186554));
#26070=DIRECTION('center_axis',(0.,0.,-1.));
#26071=DIRECTION('ref_axis',(1.,0.,0.));
#26072=DIRECTION('center_axis',(0.,0.,1.));
#26073=DIRECTION('ref_axis',(1.,0.,0.));
#26074=DIRECTION('center_axis',(0.,0.,-1.));
#26075=DIRECTION('ref_axis',(1.,0.,0.));
#26076=DIRECTION('',(0.316227766016832,3.87267321454031E-17,0.948683298050516));
#26077=DIRECTION('center_axis',(0.,0.,1.));
#26078=DIRECTION('ref_axis',(1.,0.,0.));
#26079=DIRECTION('center_axis',(0.,0.,1.));
#26080=DIRECTION('ref_axis',(1.,0.,0.));
#26081=DIRECTION('',(0.,0.,1.));
#26082=DIRECTION('center_axis',(0.,0.,1.));
#26083=DIRECTION('ref_axis',(1.,0.,0.));
#26084=DIRECTION('center_axis',(0.,0.,1.));
#26085=DIRECTION('ref_axis',(1.,0.,0.));
#26086=DIRECTION('',(-0.70710678118654,-8.65956056235484E-17,0.707106781186555));
#26087=DIRECTION('center_axis',(0.,0.,1.));
#26088=DIRECTION('ref_axis',(1.,0.,0.));
#26089=DIRECTION('center_axis',(0.,0.,-1.));
#26090=DIRECTION('ref_axis',(-1.,0.,0.));
#26091=DIRECTION('center_axis',(0.,0.,-1.));
#26092=DIRECTION('ref_axis',(1.,0.,0.));
#26093=DIRECTION('',(0.316227766016832,3.87267321454031E-17,0.948683298050516));
#26094=DIRECTION('center_axis',(0.,0.,1.));
#26095=DIRECTION('ref_axis',(1.,0.,0.));
#26096=DIRECTION('center_axis',(0.,0.,1.));
#26097=DIRECTION('ref_axis',(1.,0.,0.));
#26098=DIRECTION('',(0.,0.,1.));
#26099=DIRECTION('center_axis',(0.,0.,1.));
#26100=DIRECTION('ref_axis',(1.,0.,0.));
#26101=DIRECTION('center_axis',(0.,0.,1.));
#26102=DIRECTION('ref_axis',(1.,0.,0.));
#26103=DIRECTION('',(-0.70710678118654,-8.65956056235484E-17,0.707106781186555));
#26104=DIRECTION('center_axis',(0.,0.,1.));
#26105=DIRECTION('ref_axis',(1.,0.,0.));
#26106=DIRECTION('center_axis',(0.,0.,-1.));
#26107=DIRECTION('ref_axis',(-1.,0.,0.));
#26108=DIRECTION('center_axis',(0.,0.,-1.));
#26109=DIRECTION('ref_axis',(1.,0.,0.));
#26110=DIRECTION('',(0.316227766016832,3.87267321454031E-17,0.948683298050516));
#26111=DIRECTION('center_axis',(0.,0.,1.));
#26112=DIRECTION('ref_axis',(1.,0.,0.));
#26113=DIRECTION('center_axis',(0.,0.,1.));
#26114=DIRECTION('ref_axis',(1.,0.,0.));
#26115=DIRECTION('',(0.,0.,1.));
#26116=DIRECTION('center_axis',(0.,0.,1.));
#26117=DIRECTION('ref_axis',(1.,0.,0.));
#26118=DIRECTION('center_axis',(0.,0.,1.));
#26119=DIRECTION('ref_axis',(1.,0.,0.));
#26120=DIRECTION('',(-0.70710678118654,-8.65956056235484E-17,0.707106781186555));
#26121=DIRECTION('center_axis',(0.,0.,1.));
#26122=DIRECTION('ref_axis',(1.,0.,0.));
#26123=DIRECTION('center_axis',(0.,0.,-1.));
#26124=DIRECTION('ref_axis',(-1.,0.,0.));
#26125=DIRECTION('center_axis',(0.,0.,-1.));
#26126=DIRECTION('ref_axis',(1.,0.,0.));
#26127=DIRECTION('',(0.316227766016832,3.87267321454031E-17,0.948683298050516));
#26128=DIRECTION('center_axis',(0.,0.,1.));
#26129=DIRECTION('ref_axis',(1.,0.,0.));
#26130=DIRECTION('center_axis',(0.,0.,1.));
#26131=DIRECTION('ref_axis',(1.,0.,0.));
#26132=DIRECTION('',(0.,0.,1.));
#26133=DIRECTION('center_axis',(0.,0.,1.));
#26134=DIRECTION('ref_axis',(1.,0.,0.));
#26135=DIRECTION('center_axis',(0.,0.,1.));
#26136=DIRECTION('ref_axis',(1.,0.,0.));
#26137=DIRECTION('',(-0.70710678118654,-8.65956056235484E-17,0.707106781186555));
#26138=DIRECTION('center_axis',(0.,0.,1.));
#26139=DIRECTION('ref_axis',(1.,0.,0.));
#26140=DIRECTION('center_axis',(0.,0.,-1.));
#26141=DIRECTION('ref_axis',(-1.,0.,0.));
#26142=DIRECTION('center_axis',(-0.707106781186549,0.,-0.707106781186546));
#26143=DIRECTION('ref_axis',(-0.707106781186546,0.,0.707106781186549));
#26144=DIRECTION('center_axis',(0.,0.,-1.));
#26145=DIRECTION('ref_axis',(0.707106781186548,0.707106781186548,0.));
#26146=DIRECTION('center_axis',(-1.,0.,0.));
#26147=DIRECTION('ref_axis',(0.,-1.,0.));
#26148=DIRECTION('',(0.,0.,1.));
#26149=DIRECTION('center_axis',(0.,0.,1.));
#26150=DIRECTION('ref_axis',(0.707106781186547,0.707106781186547,0.));
#26151=DIRECTION('',(0.,0.,1.));
#26152=DIRECTION('center_axis',(0.,0.,1.));
#26153=DIRECTION('ref_axis',(-0.707106781186547,0.707106781186547,0.));
#26154=DIRECTION('',(0.,0.,-1.));
#26155=DIRECTION('center_axis',(0.,1.,0.));
#26156=DIRECTION('ref_axis',(-1.,0.,0.));
#31816=CARTESIAN_POINT('',(0.,0.,0.));
#31817=CARTESIAN_POINT('Origin',(-5.9,-4.15,1.1893933982822));
#31818=CARTESIAN_POINT('',(-6.37,-4.15,1.2));
#31819=CARTESIAN_POINT('',(-6.4212132034356,-4.15,1.1787867965644));
#31820=CARTESIAN_POINT('',(-6.37,-4.15,1.2));
#31821=CARTESIAN_POINT('',(-5.9,-4.6712132034356,1.1787867965644));
#31822=CARTESIAN_POINT('Origin',(-5.9,-4.15,1.1787867965644));
#31823=CARTESIAN_POINT('',(-5.9,-4.62,1.2));
#31824=CARTESIAN_POINT('',(-5.9,-4.6712132034356,1.1787867965644));
#31825=CARTESIAN_POINT('Origin',(-5.9,-4.15,1.2));
#31826=CARTESIAN_POINT('Origin',(-6.3956066017178,1.1875,1.1893933982822));
#31827=CARTESIAN_POINT('',(-6.37,4.15,1.2));
#31828=CARTESIAN_POINT('',(-6.4212132034356,4.15,1.1787867965644));
#31829=CARTESIAN_POINT('',(-6.37,4.15,1.2));
#31830=CARTESIAN_POINT('',(-6.4212132034356,1.1875,1.1787867965644));
#31831=CARTESIAN_POINT('',(-6.37,1.1875,1.2));
#31832=CARTESIAN_POINT('Origin',(-5.9,4.15,1.1893933982822));
#31833=CARTESIAN_POINT('',(-5.9,4.62,1.2));
#31834=CARTESIAN_POINT('',(-5.9,4.6712132034356,1.1787867965644));
#31835=CARTESIAN_POINT('',(-5.9,4.62,1.2));
#31836=CARTESIAN_POINT('Origin',(-5.9,4.15,1.1787867965644));
#31837=CARTESIAN_POINT('Origin',(-5.9,4.15,1.2));
#31838=CARTESIAN_POINT('Origin',(1.625,4.6456066017178,1.1893933982822));
#31839=CARTESIAN_POINT('',(5.9,4.62,1.2));
#31840=CARTESIAN_POINT('',(5.9,4.6712132034356,1.1787867965644));
#31841=CARTESIAN_POINT('',(5.9,4.62,1.2));
#31842=CARTESIAN_POINT('',(1.625,4.6712132034356,1.1787867965644));
#31843=CARTESIAN_POINT('',(1.625,4.62,1.2));
#31844=CARTESIAN_POINT('Origin',(5.9,4.15,1.1893933982822));
#31845=CARTESIAN_POINT('',(6.37,4.15,1.2));
#31846=CARTESIAN_POINT('',(6.4212132034356,4.15,1.1787867965644));
#31847=CARTESIAN_POINT('',(6.37,4.15,1.2));
#31848=CARTESIAN_POINT('Origin',(5.9,4.15,1.1787867965644));
#31849=CARTESIAN_POINT('Origin',(5.9,4.15,1.2));
#31850=CARTESIAN_POINT('Origin',(6.3956066017178,-1.1875,1.1893933982822));
#31851=CARTESIAN_POINT('',(6.37,-4.15,1.2));
#31852=CARTESIAN_POINT('',(6.4212132034356,-4.15,1.1787867965644));
#31853=CARTESIAN_POINT('',(6.37,-4.15,1.2));
#31854=CARTESIAN_POINT('',(6.4212132034356,-1.1875,1.1787867965644));
#31855=CARTESIAN_POINT('',(6.37,-1.1875,1.2));
#31856=CARTESIAN_POINT('Origin',(5.9,-4.15,1.1893933982822));
#31857=CARTESIAN_POINT('',(5.9,-4.62,1.2));
#31858=CARTESIAN_POINT('',(5.9,-4.6712132034356,1.1787867965644));
#31859=CARTESIAN_POINT('',(5.9,-4.62,1.2));
#31860=CARTESIAN_POINT('Origin',(5.9,-4.15,1.1787867965644));
#31861=CARTESIAN_POINT('Origin',(5.9,-4.15,1.2));
#31862=CARTESIAN_POINT('Origin',(-1.625,-4.6456066017178,1.1893933982822));
#31863=CARTESIAN_POINT('',(-1.625,-4.6712132034356,1.1787867965644));
#31864=CARTESIAN_POINT('',(-1.625,-4.62,1.2));
#31865=CARTESIAN_POINT('Origin',(6.45,-2.375,1.15));
#31866=CARTESIAN_POINT('',(6.4787867965644,-4.15,1.1212132034356));
#31867=CARTESIAN_POINT('',(6.4,-4.15,1.2));
#31868=CARTESIAN_POINT('',(6.4787867965644,4.15,1.1212132034356));
#31869=CARTESIAN_POINT('',(6.4787867965644,-3.5625,1.1212132034356));
#31870=CARTESIAN_POINT('',(6.4,4.15,1.2));
#31871=CARTESIAN_POINT('Origin',(5.9,-4.15,1.15));
#31872=CARTESIAN_POINT('',(5.9,-4.7287867965644,1.1212132034356));
#31873=CARTESIAN_POINT('',(5.9,-4.65,1.2));
#31874=CARTESIAN_POINT('Origin',(5.9,-4.15,1.1212132034356));
#31875=CARTESIAN_POINT('Origin',(-3.25,-4.7,1.15));
#31876=CARTESIAN_POINT('',(-5.9,-4.7287867965644,1.1212132034356));
#31877=CARTESIAN_POINT('',(-5.9,-4.75,1.1));
#31878=CARTESIAN_POINT('',(-4.875,-4.7287867965644,1.1212132034356));
#31879=CARTESIAN_POINT('Origin',(-5.9,-4.15,1.15));
#31880=CARTESIAN_POINT('',(-6.4787867965644,-4.15,1.1212132034356));
#31881=CARTESIAN_POINT('',(-6.4,-4.15,1.2));
#31882=CARTESIAN_POINT('Origin',(-5.9,-4.15,1.1212132034356));
#31883=CARTESIAN_POINT('Origin',(0.,0.,1.2));
#31884=CARTESIAN_POINT('',(-4.92,-3.75,1.2));
#31885=CARTESIAN_POINT('Origin',(-5.5,-3.75,1.2));
#31886=CARTESIAN_POINT('',(-4.92,3.9,1.2));
#31887=CARTESIAN_POINT('Origin',(-5.5,3.9,1.2));
#31888=CARTESIAN_POINT('',(-4.21666666666667,2.3,1.2));
#31889=CARTESIAN_POINT('Origin',(-4.5,2.3,1.2));
#31890=CARTESIAN_POINT('',(0.283333333333333,2.3,1.2));
#31891=CARTESIAN_POINT('Origin',(0.,2.3,1.2));
#31892=CARTESIAN_POINT('',(4.78333333333333,2.3,1.2));
#31893=CARTESIAN_POINT('Origin',(4.5,2.3,1.2));
#31894=CARTESIAN_POINT('',(6.08,3.9,1.2));
#31895=CARTESIAN_POINT('Origin',(5.5,3.9,1.2));
#31896=CARTESIAN_POINT('',(6.08,-3.75,1.2));
#31897=CARTESIAN_POINT('Origin',(5.5,-3.75,1.2));
#31898=CARTESIAN_POINT('Origin',(-5.9,-4.15,1.0956066017178));
#31899=CARTESIAN_POINT('',(-5.9,-4.75,1.07));
#31900=CARTESIAN_POINT('',(-5.9,-4.75,1.07));
#31901=CARTESIAN_POINT('',(-6.5,-4.15,1.07));
#31902=CARTESIAN_POINT('',(-6.4787867965644,-4.15,1.1212132034356));
#31903=CARTESIAN_POINT('Origin',(-5.9,-4.15,1.07));
#31904=CARTESIAN_POINT('Origin',(-4.875,-4.7393933982822,1.0956066017178));
#31905=CARTESIAN_POINT('',(5.9,-4.75,1.07));
#31906=CARTESIAN_POINT('',(5.9,-4.75,1.07));
#31907=CARTESIAN_POINT('',(-4.875,-4.75,1.07));
#31908=CARTESIAN_POINT('Origin',(5.9,-4.15,1.0956066017178));
#31909=CARTESIAN_POINT('',(6.5,-4.15,1.07));
#31910=CARTESIAN_POINT('',(6.5,-4.15,1.07));
#31911=CARTESIAN_POINT('Origin',(5.9,-4.15,1.07));
#31912=CARTESIAN_POINT('Origin',(6.4893933982822,-3.5625,1.0956066017178));
#31913=CARTESIAN_POINT('',(6.5,4.15,1.07));
#31914=CARTESIAN_POINT('',(6.5,4.15,1.07));
#31915=CARTESIAN_POINT('',(6.5,-3.5625,1.07));
#31916=CARTESIAN_POINT('Origin',(5.9,4.15,1.0956066017178));
#31917=CARTESIAN_POINT('',(5.9,4.75,1.07));
#31918=CARTESIAN_POINT('',(5.9,4.7287867965644,1.1212132034356));
#31919=CARTESIAN_POINT('',(5.9,4.75,1.07));
#31920=CARTESIAN_POINT('Origin',(5.9,4.15,1.1212132034356));
#31921=CARTESIAN_POINT('Origin',(5.9,4.15,1.07));
#31922=CARTESIAN_POINT('Origin',(4.875,4.7393933982822,1.0956066017178));
#31923=CARTESIAN_POINT('',(-5.9,4.75,1.07));
#31924=CARTESIAN_POINT('',(-5.9,4.7287867965644,1.1212132034356));
#31925=CARTESIAN_POINT('',(-5.9,4.75,1.07));
#31926=CARTESIAN_POINT('',(4.875,4.7287867965644,1.1212132034356));
#31927=CARTESIAN_POINT('',(4.875,4.75,1.07));
#31928=CARTESIAN_POINT('Origin',(-5.9,4.15,1.0956066017178));
#31929=CARTESIAN_POINT('',(-6.5,4.15,1.07));
#31930=CARTESIAN_POINT('',(-6.4787867965644,4.15,1.1212132034356));
#31931=CARTESIAN_POINT('',(-6.5,4.15,1.07));
#31932=CARTESIAN_POINT('Origin',(-5.9,4.15,1.1212132034356));
#31933=CARTESIAN_POINT('Origin',(-5.9,4.15,1.07));
#31934=CARTESIAN_POINT('Origin',(-6.4893933982822,3.5625,1.0956066017178));
#31935=CARTESIAN_POINT('',(-6.4787867965644,3.5625,1.1212132034356));
#31936=CARTESIAN_POINT('',(-6.5,3.5625,1.07));
#31937=CARTESIAN_POINT('Origin',(6.5,-4.75,0.));
#31938=CARTESIAN_POINT('',(6.5,-4.15,0.0800000000000016));
#31939=CARTESIAN_POINT('',(6.5,-4.15,0.));
#31940=CARTESIAN_POINT('',(6.5,4.15,0.0800000000000016));
#31941=CARTESIAN_POINT('',(6.5,-3.5625,0.0800000000000016));
#31942=CARTESIAN_POINT('',(6.5,4.15,0.));
#31943=CARTESIAN_POINT('Origin',(5.9,-4.15,0.));
#31944=CARTESIAN_POINT('',(5.9,-4.75,0.08));
#31945=CARTESIAN_POINT('',(5.9,-4.75,0.));
#31946=CARTESIAN_POINT('Origin',(5.9,-4.15,0.08));
#31947=CARTESIAN_POINT('Origin',(-6.5,-4.75,0.));
#31948=CARTESIAN_POINT('',(-5.9,-4.75,0.0800000000000016));
#31949=CARTESIAN_POINT('',(-5.9,-4.75,0.));
#31950=CARTESIAN_POINT('',(-4.875,-4.75,0.0800000000000016));
#31951=CARTESIAN_POINT('Origin',(-5.9,-4.15,0.));
#31952=CARTESIAN_POINT('',(-6.5,-4.15,0.08));
#31953=CARTESIAN_POINT('',(-6.5,-4.15,0.));
#31954=CARTESIAN_POINT('Origin',(-5.9,-4.15,0.08));
#31955=CARTESIAN_POINT('Origin',(3.25,4.7,1.15));
#31956=CARTESIAN_POINT('',(5.9,4.65,1.2));
#31957=CARTESIAN_POINT('',(-5.9,4.65,1.2));
#31958=CARTESIAN_POINT('Origin',(-5.9,4.15,1.15));
#31959=CARTESIAN_POINT('',(-6.4,4.15,1.2));
#31960=CARTESIAN_POINT('Origin',(-6.45,2.375,1.15));
#31961=CARTESIAN_POINT('Origin',(6.4456066017178,-1.1875,0.0106066017177982));
#31962=CARTESIAN_POINT('',(6.42,4.15,0.));
#31963=CARTESIAN_POINT('',(6.4712132034356,4.15,0.0212132034355961));
#31964=CARTESIAN_POINT('',(6.42,4.15,0.));
#31965=CARTESIAN_POINT('',(6.4712132034356,-4.15,0.0212132034355961));
#31966=CARTESIAN_POINT('',(6.4712132034356,-1.1875,0.0212132034355963));
#31967=CARTESIAN_POINT('',(6.42,-4.15,0.));
#31968=CARTESIAN_POINT('',(6.4712132034356,-4.15,0.0212132034355961));
#31969=CARTESIAN_POINT('',(6.42,-1.1875,0.));
#31970=CARTESIAN_POINT('Origin',(5.9,4.15,0.0106066017177981));
#31971=CARTESIAN_POINT('',(5.9,4.67,0.));
#31972=CARTESIAN_POINT('',(5.9,4.7212132034356,0.0212132034355954));
#31973=CARTESIAN_POINT('',(5.9,4.67,0.));
#31974=CARTESIAN_POINT('Origin',(5.9,4.15,0.0212132034355961));
#31975=CARTESIAN_POINT('Origin',(5.9,4.15,0.));
#31976=CARTESIAN_POINT('Origin',(1.625,4.6956066017178,0.0106066017177982));
#31977=CARTESIAN_POINT('',(-5.9,4.67,0.));
#31978=CARTESIAN_POINT('',(-5.9,4.7212132034356,0.0212132034355962));
#31979=CARTESIAN_POINT('',(-5.9,4.67,0.));
#31980=CARTESIAN_POINT('',(1.625,4.7212132034356,0.0212132034355964));
#31981=CARTESIAN_POINT('',(1.625,4.67,0.));
#31982=CARTESIAN_POINT('Origin',(-5.9,4.15,0.0106066017177981));
#31983=CARTESIAN_POINT('',(-6.42,4.15,0.));
#31984=CARTESIAN_POINT('',(-6.4712132034356,4.15,0.0212132034355954));
#31985=CARTESIAN_POINT('',(-6.42,4.15,0.));
#31986=CARTESIAN_POINT('Origin',(-5.9,4.15,0.0212132034355961));
#31987=CARTESIAN_POINT('Origin',(-5.9,4.15,0.));
#31988=CARTESIAN_POINT('Origin',(-6.4456066017178,1.1875,0.0106066017177982));
#31989=CARTESIAN_POINT('',(-6.42,-4.15,0.));
#31990=CARTESIAN_POINT('',(-6.4712132034356,-4.15,0.0212132034355961));
#31991=CARTESIAN_POINT('',(-6.42,-4.15,0.));
#31992=CARTESIAN_POINT('',(-6.4712132034356,1.1875,0.0212132034355963));
#31993=CARTESIAN_POINT('',(-6.42,1.1875,0.));
#31994=CARTESIAN_POINT('Origin',(-5.9,-4.15,0.0106066017177981));
#31995=CARTESIAN_POINT('',(-5.9,-4.67,0.));
#31996=CARTESIAN_POINT('',(-5.9,-4.7212132034356,0.0212132034355954));
#31997=CARTESIAN_POINT('',(-5.9,-4.67,0.));
#31998=CARTESIAN_POINT('Origin',(-5.9,-4.15,0.0212132034355961));
#31999=CARTESIAN_POINT('Origin',(-5.9,-4.15,0.));
#32000=CARTESIAN_POINT('Origin',(-1.625,-4.6956066017178,0.0106066017177982));
#32001=CARTESIAN_POINT('',(5.9,-4.67,0.));
#32002=CARTESIAN_POINT('',(5.9,-4.7212132034356,0.0212132034355962));
#32003=CARTESIAN_POINT('',(5.9,-4.67,0.));
#32004=CARTESIAN_POINT('',(-1.625,-4.7212132034356,0.0212132034355964));
#32005=CARTESIAN_POINT('',(-1.625,-4.67,0.));
#32006=CARTESIAN_POINT('Origin',(5.9,-4.15,0.0106066017177981));
#32007=CARTESIAN_POINT('Origin',(5.9,-4.15,0.0212132034355961));
#32008=CARTESIAN_POINT('Origin',(5.9,-4.15,0.));
#32009=CARTESIAN_POINT('Origin',(-5.9,-4.15,0.025));
#32010=CARTESIAN_POINT('',(-5.9,-4.72878679656441,0.0287867965644042));
#32011=CARTESIAN_POINT('',(-5.9,-4.7,0.));
#32012=CARTESIAN_POINT('',(-6.4787867965644,-4.15,0.0287867965644041));
#32013=CARTESIAN_POINT('Origin',(-5.9,-4.15,0.0287867965644037));
#32014=CARTESIAN_POINT('',(-6.45,-4.15,0.));
#32015=CARTESIAN_POINT('Origin',(-3.25,-4.725,0.025));
#32016=CARTESIAN_POINT('',(5.9,-4.7287867965644,0.0287867965644041));
#32017=CARTESIAN_POINT('',(5.9,-4.7,0.));
#32018=CARTESIAN_POINT('',(-4.875,-4.7287867965644,0.0287867965644046));
#32019=CARTESIAN_POINT('Origin',(5.9,-4.15,0.025));
#32020=CARTESIAN_POINT('',(6.4787867965644,-4.15,0.0287867965644044));
#32021=CARTESIAN_POINT('',(6.5,-4.15,0.05));
#32022=CARTESIAN_POINT('Origin',(5.9,-4.15,0.0287867965644037));
#32023=CARTESIAN_POINT('Origin',(6.475,-2.375,0.025));
#32024=CARTESIAN_POINT('',(6.4787867965644,4.15,0.0287867965644044));
#32025=CARTESIAN_POINT('',(6.45,4.15,0.));
#32026=CARTESIAN_POINT('',(6.4787867965644,-3.5625,0.0287867965644046));
#32027=CARTESIAN_POINT('Origin',(0.,0.,0.));
#32028=CARTESIAN_POINT('',(-5.03,2.3,0.));
#32029=CARTESIAN_POINT('Origin',(-4.5,2.3,0.));
#32030=CARTESIAN_POINT('',(3.97,2.3,0.));
#32031=CARTESIAN_POINT('Origin',(4.5,2.3,0.));
#32032=CARTESIAN_POINT('',(5.16166666666667,3.9,0.));
#32033=CARTESIAN_POINT('Origin',(5.5,3.9,0.));
#32034=CARTESIAN_POINT('',(-5.83833333333333,3.9,0.));
#32035=CARTESIAN_POINT('Origin',(-5.5,3.9,0.));
#32036=CARTESIAN_POINT('',(5.16166666666667,-3.75,0.));
#32037=CARTESIAN_POINT('Origin',(5.5,-3.75,0.));
#32038=CARTESIAN_POINT('',(-5.83833333333333,-3.75,0.));
#32039=CARTESIAN_POINT('Origin',(-5.5,-3.75,0.));
#32040=CARTESIAN_POINT('',(-0.53,2.3,0.));
#32041=CARTESIAN_POINT('Origin',(0.,2.3,0.));
#32042=CARTESIAN_POINT('Origin',(6.4893933982822,-3.5625,0.0543933982822031));
#32043=CARTESIAN_POINT('',(6.5,-4.15,0.0800000000000016));
#32044=CARTESIAN_POINT('',(6.4787867965644,4.15,0.0287867965644044));
#32045=CARTESIAN_POINT('Origin',(5.9,-4.15,0.0543933982822019));
#32046=CARTESIAN_POINT('',(5.9,-4.75,0.08));
#32047=CARTESIAN_POINT('Origin',(-4.875,-4.7393933982822,0.0543933982822031));
#32048=CARTESIAN_POINT('',(-5.9,-4.75,0.0800000000000016));
#32049=CARTESIAN_POINT('Origin',(-5.9,-4.15,0.0543933982822019));
#32050=CARTESIAN_POINT('',(-6.5,-4.15,0.08));
#32051=CARTESIAN_POINT('Origin',(-6.4893933982822,3.5625,0.0543933982822031));
#32052=CARTESIAN_POINT('',(-6.5,4.15,0.0800000000000016));
#32053=CARTESIAN_POINT('',(-6.47878679656441,4.15,0.0287867965644042));
#32054=CARTESIAN_POINT('',(-6.5,4.15,0.0800000000000016));
#32055=CARTESIAN_POINT('',(-6.4787867965644,3.5625,0.0287867965644046));
#32056=CARTESIAN_POINT('',(-6.5,3.5625,0.0800000000000016));
#32057=CARTESIAN_POINT('Origin',(-5.9,4.15,0.0543933982822019));
#32058=CARTESIAN_POINT('',(-5.9,4.75,0.08));
#32059=CARTESIAN_POINT('',(-5.9,4.7287867965644,0.0287867965644041));
#32060=CARTESIAN_POINT('',(-5.9,4.75,0.08));
#32061=CARTESIAN_POINT('Origin',(-5.9,4.15,0.0287867965644037));
#32062=CARTESIAN_POINT('Origin',(-5.9,4.15,0.08));
#32063=CARTESIAN_POINT('Origin',(4.875,4.7393933982822,0.0543933982822031));
#32064=CARTESIAN_POINT('',(5.9,4.75,0.0800000000000016));
#32065=CARTESIAN_POINT('',(5.9,4.72878679656441,0.0287867965644042));
#32066=CARTESIAN_POINT('',(5.9,4.75,0.0800000000000016));
#32067=CARTESIAN_POINT('',(4.875,4.7287867965644,0.0287867965644046));
#32068=CARTESIAN_POINT('',(4.875,4.75,0.0800000000000016));
#32069=CARTESIAN_POINT('Origin',(5.9,4.15,0.0543933982822019));
#32070=CARTESIAN_POINT('Origin',(5.9,4.15,0.0287867965644037));
#32071=CARTESIAN_POINT('Origin',(5.9,4.15,0.08));
#32072=CARTESIAN_POINT('Origin',(-5.9,4.15,0.025));
#32073=CARTESIAN_POINT('',(-6.45,4.15,0.));
#32074=CARTESIAN_POINT('',(-5.9,4.7,0.));
#32075=CARTESIAN_POINT('Origin',(3.25,4.725,0.025));
#32076=CARTESIAN_POINT('',(5.9,4.7,0.));
#32077=CARTESIAN_POINT('Origin',(5.9,4.15,0.025));
#32078=CARTESIAN_POINT('Origin',(-5.5,-3.75,1.185));
#32079=CARTESIAN_POINT('',(-4.95,-3.75,1.17));
#32080=CARTESIAN_POINT('',(-4.935,-3.75,1.185));
#32081=CARTESIAN_POINT('',(-6.05,-3.75,1.17));
#32082=CARTESIAN_POINT('Origin',(-5.5,-3.75,1.17));
#32083=CARTESIAN_POINT('Origin',(-5.5,-3.75,1.17));
#32084=CARTESIAN_POINT('Origin',(-5.5,-3.75,0.875));
#32085=CARTESIAN_POINT('',(-6.05,-3.75,0.55));
#32086=CARTESIAN_POINT('Origin',(-5.5,-3.75,0.55));
#32087=CARTESIAN_POINT('',(-6.05,-3.75,0.875));
#32088=CARTESIAN_POINT('Origin',(5.5,-3.75,1.185));
#32089=CARTESIAN_POINT('',(6.05,-3.75,1.17));
#32090=CARTESIAN_POINT('',(6.065,-3.75,1.185));
#32091=CARTESIAN_POINT('',(4.95,-3.75,1.17));
#32092=CARTESIAN_POINT('Origin',(5.5,-3.75,1.17));
#32093=CARTESIAN_POINT('Origin',(5.5,-3.75,1.17));
#32094=CARTESIAN_POINT('Origin',(5.5,-3.75,0.875));
#32095=CARTESIAN_POINT('',(4.95,-3.75,0.55));
#32096=CARTESIAN_POINT('Origin',(5.5,-3.75,0.55));
#32097=CARTESIAN_POINT('',(4.95,-3.75,0.875));
#32098=CARTESIAN_POINT('Origin',(-5.5,3.9,1.185));
#32099=CARTESIAN_POINT('',(-4.95,3.9,1.17));
#32100=CARTESIAN_POINT('',(-4.935,3.9,1.185));
#32101=CARTESIAN_POINT('',(-6.05,3.9,1.17));
#32102=CARTESIAN_POINT('Origin',(-5.5,3.9,1.17));
#32103=CARTESIAN_POINT('Origin',(-5.5,3.9,1.17));
#32104=CARTESIAN_POINT('Origin',(-5.5,3.9,0.875));
#32105=CARTESIAN_POINT('',(-6.05,3.9,0.55));
#32106=CARTESIAN_POINT('Origin',(-5.5,3.9,0.55));
#32107=CARTESIAN_POINT('',(-6.05,3.9,0.875));
#32108=CARTESIAN_POINT('Origin',(5.5,3.9,1.185));
#32109=CARTESIAN_POINT('',(6.05,3.9,1.17));
#32110=CARTESIAN_POINT('',(6.065,3.9,1.185));
#32111=CARTESIAN_POINT('',(4.95,3.9,1.17));
#32112=CARTESIAN_POINT('Origin',(5.5,3.9,1.17));
#32113=CARTESIAN_POINT('Origin',(5.5,3.9,1.17));
#32114=CARTESIAN_POINT('Origin',(5.5,3.9,0.875));
#32115=CARTESIAN_POINT('',(4.95,3.9,0.55));
#32116=CARTESIAN_POINT('Origin',(5.5,3.9,0.55));
#32117=CARTESIAN_POINT('',(4.95,3.9,0.875));
#32118=CARTESIAN_POINT('Origin',(-4.5,2.3,0.015));
#32119=CARTESIAN_POINT('',(-5.,2.3,0.03));
#32120=CARTESIAN_POINT('',(-5.015,2.3,0.015));
#32121=CARTESIAN_POINT('',(-4.,2.3,0.03));
#32122=CARTESIAN_POINT('Origin',(-4.5,2.3,0.03));
#32123=CARTESIAN_POINT('Origin',(-4.5,2.3,0.03));
#32124=CARTESIAN_POINT('Origin',(-4.5,2.3,0.275));
#32125=CARTESIAN_POINT('',(-4.,2.3,0.55));
#32126=CARTESIAN_POINT('Origin',(-4.5,2.3,0.55));
#32127=CARTESIAN_POINT('',(-4.,2.3,0.275));
#32128=CARTESIAN_POINT('Origin',(0.,2.3,0.015));
#32129=CARTESIAN_POINT('',(-0.5,2.3,0.03));
#32130=CARTESIAN_POINT('',(-0.515,2.3,0.015));
#32131=CARTESIAN_POINT('',(0.5,2.3,0.03));
#32132=CARTESIAN_POINT('Origin',(0.,2.3,0.03));
#32133=CARTESIAN_POINT('Origin',(0.,2.3,0.03));
#32134=CARTESIAN_POINT('Origin',(0.,2.3,0.275));
#32135=CARTESIAN_POINT('',(0.5,2.3,0.55));
#32136=CARTESIAN_POINT('Origin',(0.,2.3,0.55));
#32137=CARTESIAN_POINT('',(0.5,2.3,0.275));
#32138=CARTESIAN_POINT('Origin',(4.5,2.3,0.015));
#32139=CARTESIAN_POINT('',(4.,2.3,0.03));
#32140=CARTESIAN_POINT('',(3.985,2.3,0.015));
#32141=CARTESIAN_POINT('',(5.,2.3,0.03));
#32142=CARTESIAN_POINT('Origin',(4.5,2.3,0.03));
#32143=CARTESIAN_POINT('Origin',(4.5,2.3,0.03));
#32144=CARTESIAN_POINT('Origin',(4.5,2.3,0.275));
#32145=CARTESIAN_POINT('',(5.,2.3,0.55));
#32146=CARTESIAN_POINT('Origin',(4.5,2.3,0.55));
#32147=CARTESIAN_POINT('',(5.,2.3,0.275));
#32148=CARTESIAN_POINT('Origin',(4.5,2.3,1.2125));
#32149=CARTESIAN_POINT('',(4.775,2.3,1.175));
#32150=CARTESIAN_POINT('',(4.7875,2.3,1.2125));
#32151=CARTESIAN_POINT('Origin',(4.5,2.3,1.175));
#32152=CARTESIAN_POINT('Origin',(4.5,2.3,0.875));
#32153=CARTESIAN_POINT('',(4.775,2.3,0.575));
#32154=CARTESIAN_POINT('',(4.775,2.3,0.875));
#32155=CARTESIAN_POINT('Origin',(4.5,2.3,0.575));
#32156=CARTESIAN_POINT('Origin',(4.5,2.3,0.5625));
#32157=CARTESIAN_POINT('',(4.8,2.3,0.55));
#32158=CARTESIAN_POINT('',(4.7875,2.3,0.5625));
#32159=CARTESIAN_POINT('Origin',(4.5,2.3,0.55));
#32160=CARTESIAN_POINT('Origin',(4.,2.3,0.55));
#32161=CARTESIAN_POINT('Origin',(0.,2.3,1.2125));
#32162=CARTESIAN_POINT('',(0.275,2.3,1.175));
#32163=CARTESIAN_POINT('',(0.2875,2.3,1.2125));
#32164=CARTESIAN_POINT('Origin',(0.,2.3,1.175));
#32165=CARTESIAN_POINT('Origin',(0.,2.3,0.875));
#32166=CARTESIAN_POINT('',(0.275,2.3,0.575));
#32167=CARTESIAN_POINT('',(0.275,2.3,0.875));
#32168=CARTESIAN_POINT('Origin',(0.,2.3,0.575));
#32169=CARTESIAN_POINT('Origin',(0.,2.3,0.5625));
#32170=CARTESIAN_POINT('',(0.3,2.3,0.55));
#32171=CARTESIAN_POINT('',(0.2875,2.3,0.5625));
#32172=CARTESIAN_POINT('Origin',(0.,2.3,0.55));
#32173=CARTESIAN_POINT('Origin',(-0.5,2.3,0.55));
#32174=CARTESIAN_POINT('Origin',(-4.5,2.3,1.2125));
#32175=CARTESIAN_POINT('',(-4.225,2.3,1.175));
#32176=CARTESIAN_POINT('',(-4.2125,2.3,1.2125));
#32177=CARTESIAN_POINT('Origin',(-4.5,2.3,1.175));
#32178=CARTESIAN_POINT('Origin',(-4.5,2.3,0.875));
#32179=CARTESIAN_POINT('',(-4.225,2.3,0.575));
#32180=CARTESIAN_POINT('',(-4.225,2.3,0.875));
#32181=CARTESIAN_POINT('Origin',(-4.5,2.3,0.575));
#32182=CARTESIAN_POINT('Origin',(-4.5,2.3,0.5625));
#32183=CARTESIAN_POINT('',(-4.2,2.3,0.55));
#32184=CARTESIAN_POINT('',(-4.2125,2.3,0.5625));
#32185=CARTESIAN_POINT('Origin',(-4.5,2.3,0.55));
#32186=CARTESIAN_POINT('Origin',(-5.,2.3,0.55));
#32187=CARTESIAN_POINT('Origin',(5.5,3.9,-0.0125));
#32188=CARTESIAN_POINT('',(5.17,3.9,0.0249999999999998));
#32189=CARTESIAN_POINT('',(5.1575,3.9,-0.0125));
#32190=CARTESIAN_POINT('Origin',(5.5,3.9,0.0249999999999999));
#32191=CARTESIAN_POINT('Origin',(5.5,3.9,0.275));
#32192=CARTESIAN_POINT('',(5.17,3.9,0.525));
#32193=CARTESIAN_POINT('',(5.17,3.9,0.275));
#32194=CARTESIAN_POINT('Origin',(5.5,3.9,0.525));
#32195=CARTESIAN_POINT('Origin',(5.5,3.9,0.5375));
#32196=CARTESIAN_POINT('',(5.145,3.9,0.55));
#32197=CARTESIAN_POINT('',(5.1575,3.9,0.5375));
#32198=CARTESIAN_POINT('Origin',(5.5,3.9,0.55));
#32199=CARTESIAN_POINT('Origin',(6.05,3.9,0.55));
#32200=CARTESIAN_POINT('Origin',(-5.5,3.9,-0.0125));
#32201=CARTESIAN_POINT('',(-5.83,3.9,0.0249999999999998));
#32202=CARTESIAN_POINT('',(-5.8425,3.9,-0.0125));
#32203=CARTESIAN_POINT('Origin',(-5.5,3.9,0.0249999999999999));
#32204=CARTESIAN_POINT('Origin',(-5.5,3.9,0.275));
#32205=CARTESIAN_POINT('',(-5.83,3.9,0.525));
#32206=CARTESIAN_POINT('',(-5.83,3.9,0.275));
#32207=CARTESIAN_POINT('Origin',(-5.5,3.9,0.525));
#32208=CARTESIAN_POINT('Origin',(-5.5,3.9,0.5375));
#32209=CARTESIAN_POINT('',(-5.855,3.9,0.55));
#32210=CARTESIAN_POINT('',(-5.8425,3.9,0.5375));
#32211=CARTESIAN_POINT('Origin',(-5.5,3.9,0.55));
#32212=CARTESIAN_POINT('Origin',(-4.95,3.9,0.55));
#32213=CARTESIAN_POINT('Origin',(5.5,-3.75,-0.0125));
#32214=CARTESIAN_POINT('',(5.17,-3.75,0.0249999999999998));
#32215=CARTESIAN_POINT('',(5.1575,-3.75,-0.0125));
#32216=CARTESIAN_POINT('Origin',(5.5,-3.75,0.0249999999999999));
#32217=CARTESIAN_POINT('Origin',(5.5,-3.75,0.275));
#32218=CARTESIAN_POINT('',(5.17,-3.75,0.525));
#32219=CARTESIAN_POINT('',(5.17,-3.75,0.275));
#32220=CARTESIAN_POINT('Origin',(5.5,-3.75,0.525));
#32221=CARTESIAN_POINT('Origin',(5.5,-3.75,0.5375));
#32222=CARTESIAN_POINT('',(5.145,-3.75,0.55));
#32223=CARTESIAN_POINT('',(5.1575,-3.75,0.5375));
#32224=CARTESIAN_POINT('Origin',(5.5,-3.75,0.55));
#32225=CARTESIAN_POINT('Origin',(6.05,-3.75,0.55));
#32226=CARTESIAN_POINT('Origin',(-5.5,-3.75,-0.0125));
#32227=CARTESIAN_POINT('',(-5.83,-3.75,0.0249999999999998));
#32228=CARTESIAN_POINT('',(-5.8425,-3.75,-0.0125));
#32229=CARTESIAN_POINT('Origin',(-5.5,-3.75,0.0249999999999999));
#32230=CARTESIAN_POINT('Origin',(-5.5,-3.75,0.275));
#32231=CARTESIAN_POINT('',(-5.83,-3.75,0.525));
#32232=CARTESIAN_POINT('',(-5.83,-3.75,0.275));
#32233=CARTESIAN_POINT('Origin',(-5.5,-3.75,0.525));
#32234=CARTESIAN_POINT('Origin',(-5.5,-3.75,0.5375));
#32235=CARTESIAN_POINT('',(-5.855,-3.75,0.55));
#32236=CARTESIAN_POINT('',(-5.8425,-3.75,0.5375));
#32237=CARTESIAN_POINT('Origin',(-5.5,-3.75,0.55));
#32238=CARTESIAN_POINT('Origin',(-4.95,-3.75,0.55));
#32239=CARTESIAN_POINT('Origin',(-6.475,2.375,0.025));
#32240=CARTESIAN_POINT('Origin',(5.9,4.15,1.15));
#32241=CARTESIAN_POINT('Origin',(-6.5,4.75,0.));
#32242=CARTESIAN_POINT('',(-6.5,4.15,0.));
#32243=CARTESIAN_POINT('Origin',(5.9,4.15,0.));
#32244=CARTESIAN_POINT('',(5.9,4.75,0.));
#32245=CARTESIAN_POINT('Origin',(-5.9,4.15,0.));
#32246=CARTESIAN_POINT('',(-5.9,4.75,0.));
#32247=CARTESIAN_POINT('Origin',(6.5,4.75,0.));
#53616=UNCERTAINTY_MEASURE_WITH_UNIT(LENGTH_MEASURE(0.001),#53651,
'DISTANCE_ACCURACY_VALUE',
'Maximum model space distance between geometric entities at asserted c
onnectivities');
#53632=UNCERTAINTY_MEASURE_WITH_UNIT(LENGTH_MEASURE(0.001),#53651,
'DISTANCE_ACCURACY_VALUE',
'Maximum model space distance between geometric entities at asserted c
onnectivities');
#53634=(
GEOMETRIC_REPRESENTATION_CONTEXT(3)
GLOBAL_UNCERTAINTY_ASSIGNED_CONTEXT((#53616))
GLOBAL_UNIT_ASSIGNED_CONTEXT((#53651,#53653,#53654))
REPRESENTATION_CONTEXT('','3D')
);
#53650=(
GEOMETRIC_REPRESENTATION_CONTEXT(3)
GLOBAL_UNCERTAINTY_ASSIGNED_CONTEXT((#53632))
GLOBAL_UNIT_ASSIGNED_CONTEXT((#53651,#53653,#53654))
REPRESENTATION_CONTEXT('','3D')
);
#53651=(
LENGTH_UNIT()
NAMED_UNIT(*)
SI_UNIT(.CENTI.,.METRE.)
);
#53653=(
NAMED_UNIT(*)
PLANE_ANGLE_UNIT()
SI_UNIT($,.RADIAN.)
);
#53654=(
NAMED_UNIT(*)
SI_UNIT($,.STERADIAN.)
SOLID_ANGLE_UNIT()
);
#53656=SHAPE_DEFINITION_REPRESENTATION(#53673,#53724);
#53673=PRODUCT_DEFINITION_SHAPE('',$,#53742);
#53724=SHAPE_REPRESENTATION('',(#23497),#53634);
#53740=PRODUCT_DEFINITION_CONTEXT('part definition',#53793,'design');
#53742=PRODUCT_DEFINITION('2026-10-18-22-44-24-012','01_Base_Flange',#53759,
#53740);
#53759=PRODUCT_DEFINITION_FORMATION('',$,#53796);
#53793=APPLICATION_CONTEXT(
'Core Data for Automotive Mechanical Design Process');
#53794=PRODUCT_CONTEXT('part definition',#53793,'mechanical');
#53796=PRODUCT('2026-10-18-22-44-24-012','01_Base_Flange',$,(#53794));
#53931=COLOUR_RGB('Dark Blue',0.08,0.2,0.34);
#53932=FILL_AREA_STYLE_COLOUR('',#53931);
#53933=FILL_AREA_STYLE('',(#53932));
#53934=SURFACE_STYLE_FILL_AREA(#53933);
#53935=SURFACE_SIDE_STYLE('',(#53934));
#53936=SURFACE_STYLE_USAGE(.BOTH.,#53935);
#53937=PRESENTATION_STYLE_ASSIGNMENT((#53936));
ENDSEC;
END-ISO-10303-21;
